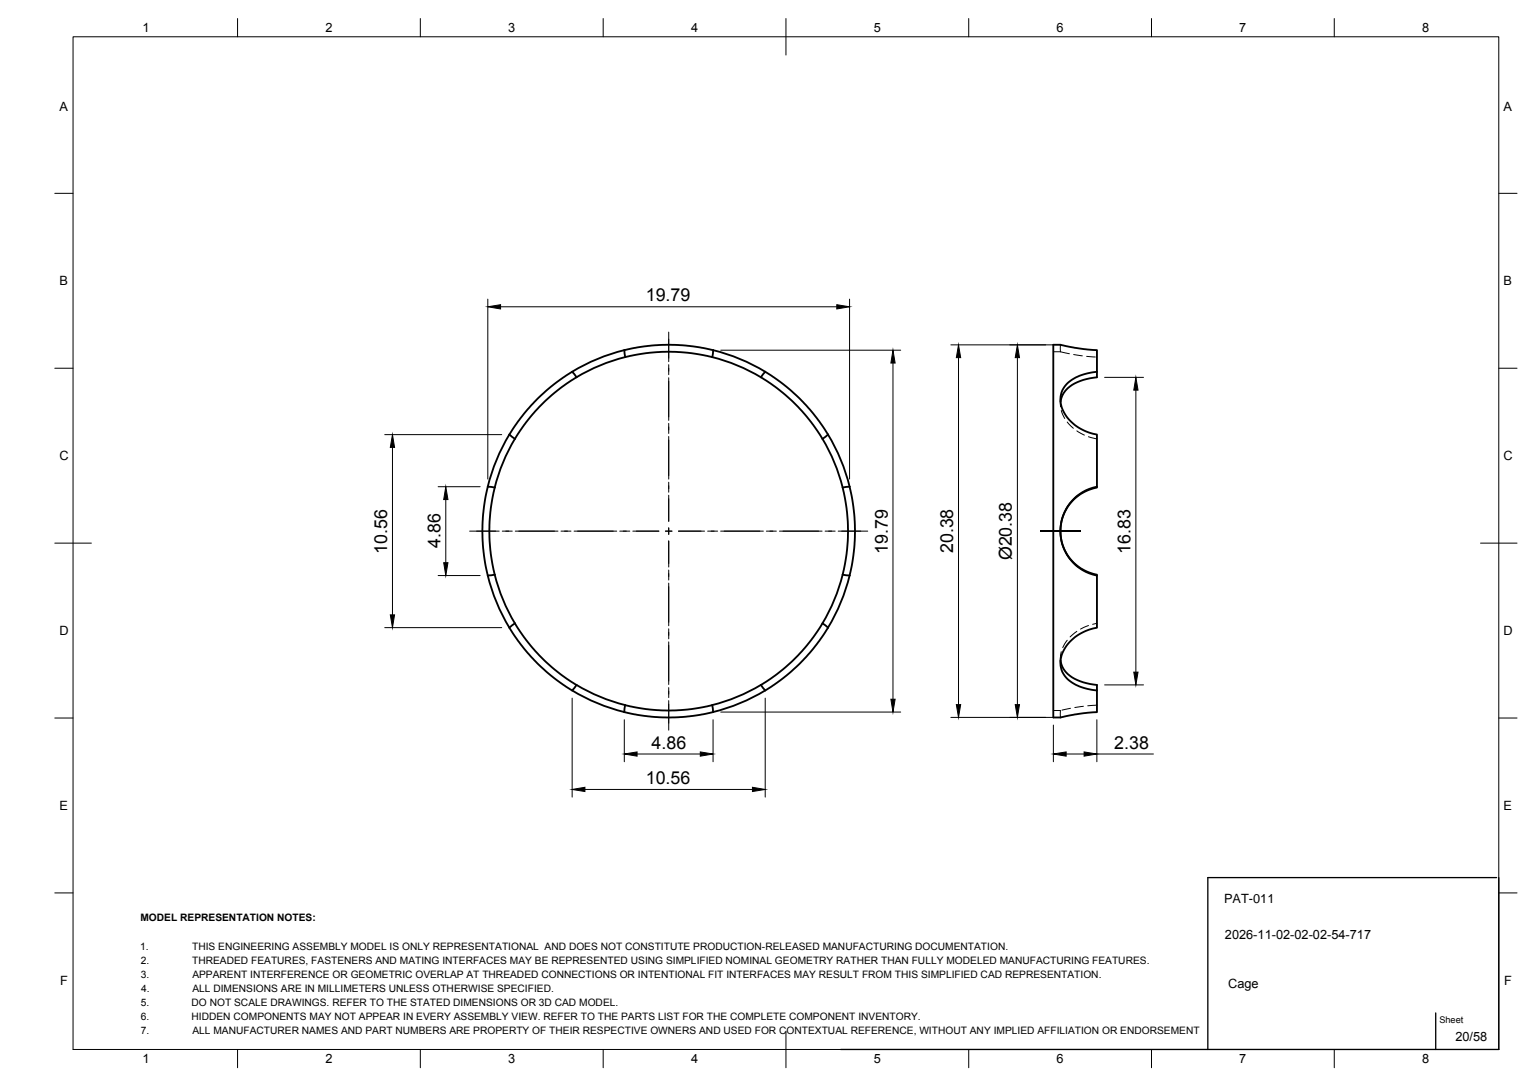
ISO-10303-21;
HEADER;
/* Generated by software containing ST-Developer
 * from STEP Tools, Inc. (www.steptools.com) 
 */

FILE_DESCRIPTION(
/* description */ ('Belt tension measurement rig'),
/* implementation_level */ '2;1');

FILE_NAME(
/* name */ 'Cage.step',
/* time_stamp */ '2026-10-28T03:24:44-07:00',
/* author */ (''),
/* organization */ (''),
/* preprocessor_version */ 'ST-DEVELOPER v20.2',
/* originating_system */ 'Autodesk Translation Framework v15.17.0.0',
/* authorisation */ '');

FILE_SCHEMA (('AUTOMOTIVE_DESIGN { 1 0 10303 214 3 1 1 }'));
ENDSEC;

DATA;
#10=MECHANICAL_DESIGN_GEOMETRIC_PRESENTATION_REPRESENTATION('',(#716),#23587);
#445=SPHERICAL_SURFACE('',#13280,0.247676);
#446=SPHERICAL_SURFACE('',#13296,0.247676);
#447=SPHERICAL_SURFACE('',#13301,0.247676);
#448=SPHERICAL_SURFACE('',#13306,0.247676);
#449=SPHERICAL_SURFACE('',#13311,0.247676);
#450=SPHERICAL_SURFACE('',#13316,0.247676);
#451=SPHERICAL_SURFACE('',#13321,0.247676);
#452=SPHERICAL_SURFACE('',#13329,0.247676);
#495=B_SPLINE_CURVE_WITH_KNOTS('',3,(#19542,#19543,#19544,#19545,#19546,
#19547,#19548,#19549,#19550,#19551,#19552,#19553,#19554,#19555,#19556,#19557,
#19558,#19559,#19560,#19561,#19562,#19563),.UNSPECIFIED.,.F.,.F.,(4,2,2,
2,2,2,2,2,2,2,4),(0.0473477652366656,0.126350602536658,0.189525903804987,
0.252701205073317,0.313298422430275,0.373895639787233,0.434492857144191,
0.495090074501149,0.558265375769478,0.621440677037807,0.7004435143378),
 .UNSPECIFIED.);
#496=B_SPLINE_CURVE_WITH_KNOTS('',3,(#19567,#19568,#19569,#19570,#19571,
#19572,#19573,#19574,#19575,#19576,#19577,#19578,#19579,#19580,#19581,#19582,
#19583,#19584,#19585,#19586,#19587,#19588),.UNSPECIFIED.,.F.,.F.,(4,2,2,
2,2,2,2,2,2,2,4),(0.0464897534940957,0.0852567806515119,0.170513561303024,
0.246687263103517,0.308657850341199,0.370628437578881,0.432599024816563,
0.494569612054245,0.570743313854739,0.656000094506251,0.694767121663666),
 .UNSPECIFIED.);
#497=B_SPLINE_CURVE_WITH_KNOTS('',3,(#19594,#19595,#19596,#19597,#19598,
#19599,#19600,#19601,#19602,#19603,#19604,#19605,#19606,#19607,#19608,#19609,
#19610,#19611,#19612,#19613,#19614,#19615),.UNSPECIFIED.,.F.,.F.,(4,2,2,
2,2,2,2,2,2,2,4),(0.0464897534940957,0.0852567806515118,0.170513561303024,
0.246687263103517,0.308657850341199,0.370628437578881,0.432599024816563,
0.494569612054245,0.570743313854738,0.65600009450625,0.694767121663666),
 .UNSPECIFIED.);
#498=B_SPLINE_CURVE_WITH_KNOTS('',3,(#19619,#19620,#19621,#19622,#19623,
#19624,#19625,#19626,#19627,#19628,#19629,#19630,#19631,#19632,#19633,#19634,
#19635,#19636,#19637,#19638,#19639,#19640),.UNSPECIFIED.,.F.,.F.,(4,2,2,
2,2,2,2,2,2,2,4),(0.0464897534940957,0.0852567806515119,0.170513561303024,
0.246687263103517,0.308657850341199,0.370628437578881,0.432599024816563,
0.494569612054245,0.570743313854739,0.656000094506251,0.694767121663666),
 .UNSPECIFIED.);
#499=B_SPLINE_CURVE_WITH_KNOTS('',3,(#19644,#19645,#19646,#19647,#19648,
#19649,#19650,#19651,#19652,#19653,#19654,#19655),.UNSPECIFIED.,.F.,.F.,
(4,2,2,2,2,4),(0.0464897534940957,0.0852567806515119,0.170513561303024,
0.246687263103517,0.308657850341199,0.370628437578881),.UNSPECIFIED.);
#500=B_SPLINE_CURVE_WITH_KNOTS('',3,(#19660,#19661,#19662,#19663,#19664,
#19665,#19666,#19667,#19668,#19669,#19670,#19671),.UNSPECIFIED.,.F.,.F.,
(4,2,2,2,2,4),(0.370628437578881,0.432599024816563,0.494569612054245,0.570743313854738,
0.65600009450625,0.694767121663666),.UNSPECIFIED.);
#501=B_SPLINE_CURVE_WITH_KNOTS('',3,(#19675,#19676,#19677,#19678,#19679,
#19680,#19681,#19682,#19683,#19684,#19685,#19686,#19687,#19688,#19689,#19690,
#19691,#19692,#19693,#19694,#19695,#19696),.UNSPECIFIED.,.F.,.F.,(4,2,2,
2,2,2,2,2,2,2,4),(0.0464897534940957,0.0852567806515121,0.170513561303024,
0.246687263103518,0.308657850341199,0.370628437578881,0.432599024816563,
0.494569612054245,0.570743313854738,0.65600009450625,0.694767121663666),
 .UNSPECIFIED.);
#502=B_SPLINE_CURVE_WITH_KNOTS('',3,(#19700,#19701,#19702,#19703,#19704,
#19705,#19706,#19707,#19708,#19709,#19710,#19711,#19712,#19713,#19714,#19715,
#19716,#19717,#19718,#19719,#19720,#19721),.UNSPECIFIED.,.F.,.F.,(4,2,2,
2,2,2,2,2,2,2,4),(0.0464897534940957,0.0852567806515119,0.170513561303024,
0.246687263103517,0.308657850341199,0.370628437578881,0.432599024816563,
0.494569612054245,0.570743313854738,0.65600009450625,0.694767121663667),
 .UNSPECIFIED.);
#503=B_SPLINE_CURVE_WITH_KNOTS('',3,(#19725,#19726,#19727,#19728,#19729,
#19730,#19731,#19732,#19733,#19734,#19735,#19736,#19737,#19738,#19739,#19740,
#19741,#19742,#19743,#19744,#19745,#19746),.UNSPECIFIED.,.F.,.F.,(4,2,2,
2,2,2,2,2,2,2,4),(0.0464897534940957,0.0852567806515119,0.170513561303024,
0.246687263103517,0.308657850341199,0.370628437578881,0.432599024816563,
0.494569612054245,0.570743313854738,0.65600009450625,0.694767121663666),
 .UNSPECIFIED.);
#504=B_SPLINE_CURVE_WITH_KNOTS('',3,(#19750,#19751,#19752,#19753,#19754,
#19755,#19756,#19757,#19758,#19759,#19760,#19761,#19762,#19763,#19764,#19765,
#19766,#19767,#19768,#19769,#19770,#19771),.UNSPECIFIED.,.F.,.F.,(4,2,2,
2,2,2,2,2,2,2,4),(0.0464897534940957,0.0852567806515119,0.170513561303024,
0.246687263103517,0.308657850341199,0.370628437578881,0.432599024816563,
0.494569612054245,0.570743313854739,0.656000094506251,0.694767121663667),
 .UNSPECIFIED.);
#505=B_SPLINE_CURVE_WITH_KNOTS('',3,(#19779,#19780,#19781,#19782,#19783,
#19784,#19785,#19786,#19787,#19788,#19789,#19790,#19791,#19792,#19793,#19794,
#19795,#19796,#19797,#19798,#19799,#19800),.UNSPECIFIED.,.F.,.F.,(4,2,2,
2,2,2,2,2,2,2,4),(0.0473477652366656,0.126350602536658,0.189525903804987,
0.252701205073316,0.313298422430274,0.373895639787232,0.434492857144191,
0.495090074501149,0.558265375769478,0.621440677037807,0.7004435143378),
 .UNSPECIFIED.);
#506=B_SPLINE_CURVE_WITH_KNOTS('',3,(#19808,#19809,#19810,#19811,#19812,
#19813,#19814,#19815,#19816,#19817,#19818,#19819,#19820,#19821,#19822,#19823,
#19824,#19825,#19826,#19827,#19828,#19829),.UNSPECIFIED.,.F.,.F.,(4,2,2,
2,2,2,2,2,2,2,4),(0.0473477652366656,0.126350602536658,0.189525903804987,
0.252701205073317,0.313298422430275,0.373895639787233,0.434492857144191,
0.495090074501149,0.558265375769478,0.621440677037807,0.7004435143378),
 .UNSPECIFIED.);
#507=B_SPLINE_CURVE_WITH_KNOTS('',3,(#19838,#19839,#19840,#19841,#19842,
#19843,#19844,#19845,#19846,#19847,#19848,#19849),.UNSPECIFIED.,.F.,.F.,
(4,2,2,2,2,4),(0.0473477652366656,0.126350602536658,0.189525903804987,0.252701205073316,
0.313298422430275,0.373895639787233),.UNSPECIFIED.);
#508=B_SPLINE_CURVE_WITH_KNOTS('',3,(#19851,#19852,#19853,#19854,#19855,
#19856,#19857,#19858,#19859,#19860,#19861,#19862),.UNSPECIFIED.,.F.,.F.,
(4,2,2,2,2,4),(0.373895639787233,0.434492857144191,0.495090074501149,0.558265375769478,
0.621440677037807,0.7004435143378),.UNSPECIFIED.);
#509=B_SPLINE_CURVE_WITH_KNOTS('',3,(#19869,#19870,#19871,#19872,#19873,
#19874,#19875,#19876,#19877,#19878,#19879,#19880,#19881,#19882,#19883,#19884,
#19885,#19886,#19887,#19888,#19889,#19890),.UNSPECIFIED.,.F.,.F.,(4,2,2,
2,2,2,2,2,2,2,4),(0.0473477652366656,0.126350602536658,0.189525903804987,
0.252701205073316,0.313298422430275,0.373895639787233,0.434492857144191,
0.495090074501149,0.558265375769478,0.621440677037807,0.7004435143378),
 .UNSPECIFIED.);
#510=B_SPLINE_CURVE_WITH_KNOTS('',3,(#19898,#19899,#19900,#19901,#19902,
#19903,#19904,#19905,#19906,#19907,#19908,#19909,#19910,#19911,#19912,#19913,
#19914,#19915,#19916,#19917,#19918,#19919),.UNSPECIFIED.,.F.,.F.,(4,2,2,
2,2,2,2,2,2,2,4),(0.0473477652366656,0.126350602536658,0.189525903804987,
0.252701205073317,0.313298422430275,0.373895639787233,0.434492857144191,
0.495090074501149,0.558265375769478,0.621440677037807,0.7004435143378),
 .UNSPECIFIED.);
#511=B_SPLINE_CURVE_WITH_KNOTS('',3,(#19927,#19928,#19929,#19930,#19931,
#19932,#19933,#19934,#19935,#19936,#19937,#19938,#19939,#19940,#19941,#19942,
#19943,#19944,#19945,#19946,#19947,#19948),.UNSPECIFIED.,.F.,.F.,(4,2,2,
2,2,2,2,2,2,2,4),(0.0473477652366656,0.126350602536658,0.189525903804987,
0.252701205073316,0.313298422430275,0.373895639787233,0.434492857144191,
0.495090074501149,0.558265375769478,0.621440677037807,0.7004435143378),
 .UNSPECIFIED.);
#512=B_SPLINE_CURVE_WITH_KNOTS('',3,(#19957,#19958,#19959,#19960,#19961,
#19962,#19963,#19964,#19965,#19966,#19967,#19968,#19969,#19970,#19971,#19972,
#19973,#19974,#19975,#19976,#19977,#19978),.UNSPECIFIED.,.F.,.F.,(4,2,2,
2,2,2,2,2,2,2,4),(0.0473477652366656,0.126350602536658,0.189525903804987,
0.252701205073317,0.313298422430275,0.373895639787233,0.434492857144191,
0.495090074501149,0.558265375769478,0.621440677037807,0.7004435143378),
 .UNSPECIFIED.);
#599=SHAPE_REPRESENTATION_RELATIONSHIP('SRR','None',#23845,#654);
#654=ADVANCED_BREP_SHAPE_REPRESENTATION('',(#786),#23543);
#716=STYLED_ITEM('',(#24211),#786);
#786=MANIFOLD_SOLID_BREP('Continuous crown cage',#12221);
#911=FACE_BOUND('',#2357,.T.);
#1142=PLANE('',#13293);
#1143=PLANE('',#13298);
#1144=PLANE('',#13303);
#1145=PLANE('',#13308);
#1146=PLANE('',#13313);
#1147=PLANE('',#13318);
#1148=PLANE('',#13327);
#1149=PLANE('',#13331);
#1150=PLANE('',#13332);
#1553=FACE_OUTER_BOUND('',#2339,.T.);
#1554=FACE_OUTER_BOUND('',#2340,.T.);
#1555=FACE_OUTER_BOUND('',#2341,.T.);
#1556=FACE_OUTER_BOUND('',#2342,.T.);
#1557=FACE_OUTER_BOUND('',#2343,.T.);
#1558=FACE_OUTER_BOUND('',#2344,.T.);
#1559=FACE_OUTER_BOUND('',#2345,.T.);
#1560=FACE_OUTER_BOUND('',#2346,.T.);
#1561=FACE_OUTER_BOUND('',#2347,.T.);
#1562=FACE_OUTER_BOUND('',#2348,.T.);
#1563=FACE_OUTER_BOUND('',#2349,.T.);
#1564=FACE_OUTER_BOUND('',#2350,.T.);
#1565=FACE_OUTER_BOUND('',#2351,.T.);
#1566=FACE_OUTER_BOUND('',#2352,.T.);
#1567=FACE_OUTER_BOUND('',#2353,.T.);
#1568=FACE_OUTER_BOUND('',#2354,.T.);
#1569=FACE_OUTER_BOUND('',#2355,.T.);
#1570=FACE_OUTER_BOUND('',#2356,.T.);
#1571=FACE_OUTER_BOUND('',#2358,.T.);
#2339=EDGE_LOOP('',(#8764,#8765,#8766,#8767));
#2340=EDGE_LOOP('',(#8768,#8769,#8770,#8771,#8772,#8773,#8774,#8775,#8776,
#8777,#8778,#8779,#8780,#8781,#8782,#8783,#8784,#8785,#8786,#8787));
#2341=EDGE_LOOP('',(#8788,#8789,#8790,#8791));
#2342=EDGE_LOOP('',(#8792,#8793,#8794,#8795));
#2343=EDGE_LOOP('',(#8796,#8797,#8798,#8799));
#2344=EDGE_LOOP('',(#8800,#8801,#8802,#8803));
#2345=EDGE_LOOP('',(#8804,#8805,#8806,#8807));
#2346=EDGE_LOOP('',(#8808,#8809,#8810,#8811,#8812,#8813));
#2347=EDGE_LOOP('',(#8814,#8815,#8816,#8817));
#2348=EDGE_LOOP('',(#8818,#8819,#8820,#8821));
#2349=EDGE_LOOP('',(#8822,#8823,#8824,#8825));
#2350=EDGE_LOOP('',(#8826,#8827,#8828,#8829));
#2351=EDGE_LOOP('',(#8830,#8831,#8832,#8833));
#2352=EDGE_LOOP('',(#8834,#8835,#8836,#8837));
#2353=EDGE_LOOP('',(#8838,#8839,#8840,#8841,#8842,#8843,#8844,#8845,#8846,
#8847,#8848,#8849,#8850,#8851,#8852,#8853,#8854,#8855,#8856,#8857));
#2354=EDGE_LOOP('',(#8858,#8859,#8860,#8861));
#2355=EDGE_LOOP('',(#8862,#8863,#8864,#8865));
#2356=EDGE_LOOP('',(#8866));
#2357=EDGE_LOOP('',(#8867));
#2358=EDGE_LOOP('',(#8868,#8869,#8870,#8871));
#3195=LINE('',#19657,#3946);
#3196=LINE('',#19953,#3947);
#3946=VECTOR('',#15566,1.019052);
#3947=VECTOR('',#15643,0.980948);
#4652=CIRCLE('',#13281,0.243053047864041);
#4653=CIRCLE('',#13282,0.243053047864041);
#4654=CIRCLE('',#13284,1.019052);
#4655=CIRCLE('',#13285,1.019052);
#4656=CIRCLE('',#13286,1.019052);
#4657=CIRCLE('',#13287,1.019052);
#4658=CIRCLE('',#13288,1.019052);
#4659=CIRCLE('',#13289,1.019052);
#4660=CIRCLE('',#13290,1.019052);
#4661=CIRCLE('',#13291,1.019052);
#4662=CIRCLE('',#13292,1.019052);
#4663=CIRCLE('',#13294,0.980948);
#4664=CIRCLE('',#13295,0.243053047864041);
#4665=CIRCLE('',#13297,0.243053047864041);
#4666=CIRCLE('',#13299,0.980948);
#4667=CIRCLE('',#13300,0.243053047864041);
#4668=CIRCLE('',#13302,0.243053047864041);
#4669=CIRCLE('',#13304,0.980948);
#4670=CIRCLE('',#13305,0.243053047864041);
#4671=CIRCLE('',#13307,0.243053047864041);
#4672=CIRCLE('',#13309,0.980948);
#4673=CIRCLE('',#13310,0.243053047864041);
#4674=CIRCLE('',#13312,0.243053047864041);
#4675=CIRCLE('',#13314,0.980948);
#4676=CIRCLE('',#13315,0.243053047864041);
#4677=CIRCLE('',#13317,0.243053047864041);
#4678=CIRCLE('',#13319,0.980948);
#4679=CIRCLE('',#13320,0.243053047864041);
#4680=CIRCLE('',#13322,0.243053047864041);
#4681=CIRCLE('',#13324,0.980948);
#4682=CIRCLE('',#13325,0.980948);
#4683=CIRCLE('',#13326,0.980948);
#4684=CIRCLE('',#13328,0.243053047864041);
#4685=CIRCLE('',#13330,0.243053047864041);
#5520=VERTEX_POINT('',#19540);
#5521=VERTEX_POINT('',#19541);
#5522=VERTEX_POINT('',#19564);
#5523=VERTEX_POINT('',#19566);
#5524=VERTEX_POINT('',#19591);
#5525=VERTEX_POINT('',#19593);
#5526=VERTEX_POINT('',#19616);
#5527=VERTEX_POINT('',#19618);
#5528=VERTEX_POINT('',#19641);
#5529=VERTEX_POINT('',#19643);
#5530=VERTEX_POINT('',#19656);
#5531=VERTEX_POINT('',#19659);
#5532=VERTEX_POINT('',#19672);
#5533=VERTEX_POINT('',#19674);
#5534=VERTEX_POINT('',#19697);
#5535=VERTEX_POINT('',#19699);
#5536=VERTEX_POINT('',#19722);
#5537=VERTEX_POINT('',#19724);
#5538=VERTEX_POINT('',#19747);
#5539=VERTEX_POINT('',#19749);
#5540=VERTEX_POINT('',#19774);
#5541=VERTEX_POINT('',#19778);
#5542=VERTEX_POINT('',#19803);
#5543=VERTEX_POINT('',#19807);
#5544=VERTEX_POINT('',#19832);
#5545=VERTEX_POINT('',#19836);
#5546=VERTEX_POINT('',#19837);
#5547=VERTEX_POINT('',#19864);
#5548=VERTEX_POINT('',#19868);
#5549=VERTEX_POINT('',#19893);
#5550=VERTEX_POINT('',#19897);
#5551=VERTEX_POINT('',#19922);
#5552=VERTEX_POINT('',#19926);
#5553=VERTEX_POINT('',#19951);
#5554=VERTEX_POINT('',#19954);
#5555=VERTEX_POINT('',#19956);
#6741=EDGE_CURVE('',#5520,#5521,#495,.T.);
#6742=EDGE_CURVE('',#5522,#5520,#4652,.T.);
#6743=EDGE_CURVE('',#5523,#5522,#496,.T.);
#6744=EDGE_CURVE('',#5521,#5523,#4653,.T.);
#6745=EDGE_CURVE('',#5524,#5522,#4654,.T.);
#6746=EDGE_CURVE('',#5524,#5525,#497,.T.);
#6747=EDGE_CURVE('',#5526,#5525,#4655,.T.);
#6748=EDGE_CURVE('',#5526,#5527,#498,.T.);
#6749=EDGE_CURVE('',#5528,#5527,#4656,.T.);
#6750=EDGE_CURVE('',#5528,#5529,#499,.T.);
#6751=EDGE_CURVE('',#5529,#5530,#3195,.T.);
#6752=EDGE_CURVE('',#5530,#5530,#4657,.T.);
#6753=EDGE_CURVE('',#5529,#5531,#500,.T.);
#6754=EDGE_CURVE('',#5532,#5531,#4658,.T.);
#6755=EDGE_CURVE('',#5532,#5533,#501,.T.);
#6756=EDGE_CURVE('',#5534,#5533,#4659,.T.);
#6757=EDGE_CURVE('',#5534,#5535,#502,.T.);
#6758=EDGE_CURVE('',#5536,#5535,#4660,.T.);
#6759=EDGE_CURVE('',#5536,#5537,#503,.T.);
#6760=EDGE_CURVE('',#5538,#5537,#4661,.T.);
#6761=EDGE_CURVE('',#5538,#5539,#504,.T.);
#6762=EDGE_CURVE('',#5523,#5539,#4662,.T.);
#6763=EDGE_CURVE('',#5520,#5540,#4663,.T.);
#6764=EDGE_CURVE('',#5540,#5524,#4664,.T.);
#6765=EDGE_CURVE('',#5541,#5540,#505,.T.);
#6766=EDGE_CURVE('',#5525,#5541,#4665,.T.);
#6767=EDGE_CURVE('',#5541,#5542,#4666,.T.);
#6768=EDGE_CURVE('',#5542,#5526,#4667,.T.);
#6769=EDGE_CURVE('',#5543,#5542,#506,.T.);
#6770=EDGE_CURVE('',#5527,#5543,#4668,.T.);
#6771=EDGE_CURVE('',#5543,#5544,#4669,.T.);
#6772=EDGE_CURVE('',#5544,#5528,#4670,.T.);
#6773=EDGE_CURVE('',#5545,#5546,#507,.T.);
#6774=EDGE_CURVE('',#5531,#5545,#4671,.T.);
#6775=EDGE_CURVE('',#5546,#5544,#508,.T.);
#6776=EDGE_CURVE('',#5545,#5547,#4672,.T.);
#6777=EDGE_CURVE('',#5547,#5532,#4673,.T.);
#6778=EDGE_CURVE('',#5548,#5547,#509,.T.);
#6779=EDGE_CURVE('',#5533,#5548,#4674,.T.);
#6780=EDGE_CURVE('',#5548,#5549,#4675,.T.);
#6781=EDGE_CURVE('',#5549,#5534,#4676,.T.);
#6782=EDGE_CURVE('',#5550,#5549,#510,.T.);
#6783=EDGE_CURVE('',#5535,#5550,#4677,.T.);
#6784=EDGE_CURVE('',#5550,#5551,#4678,.T.);
#6785=EDGE_CURVE('',#5551,#5536,#4679,.T.);
#6786=EDGE_CURVE('',#5552,#5551,#511,.T.);
#6787=EDGE_CURVE('',#5537,#5552,#4680,.T.);
#6788=EDGE_CURVE('',#5553,#5553,#4681,.T.);
#6789=EDGE_CURVE('',#5553,#5546,#3196,.T.);
#6790=EDGE_CURVE('',#5554,#5521,#4682,.T.);
#6791=EDGE_CURVE('',#5554,#5555,#512,.T.);
#6792=EDGE_CURVE('',#5552,#5555,#4683,.T.);
#6793=EDGE_CURVE('',#5539,#5554,#4684,.T.);
#6794=EDGE_CURVE('',#5555,#5538,#4685,.T.);
#8764=ORIENTED_EDGE('',*,*,#6741,.F.);
#8765=ORIENTED_EDGE('',*,*,#6742,.F.);
#8766=ORIENTED_EDGE('',*,*,#6743,.F.);
#8767=ORIENTED_EDGE('',*,*,#6744,.F.);
#8768=ORIENTED_EDGE('',*,*,#6743,.T.);
#8769=ORIENTED_EDGE('',*,*,#6745,.F.);
#8770=ORIENTED_EDGE('',*,*,#6746,.T.);
#8771=ORIENTED_EDGE('',*,*,#6747,.F.);
#8772=ORIENTED_EDGE('',*,*,#6748,.T.);
#8773=ORIENTED_EDGE('',*,*,#6749,.F.);
#8774=ORIENTED_EDGE('',*,*,#6750,.T.);
#8775=ORIENTED_EDGE('',*,*,#6751,.T.);
#8776=ORIENTED_EDGE('',*,*,#6752,.F.);
#8777=ORIENTED_EDGE('',*,*,#6751,.F.);
#8778=ORIENTED_EDGE('',*,*,#6753,.T.);
#8779=ORIENTED_EDGE('',*,*,#6754,.F.);
#8780=ORIENTED_EDGE('',*,*,#6755,.T.);
#8781=ORIENTED_EDGE('',*,*,#6756,.F.);
#8782=ORIENTED_EDGE('',*,*,#6757,.T.);
#8783=ORIENTED_EDGE('',*,*,#6758,.F.);
#8784=ORIENTED_EDGE('',*,*,#6759,.T.);
#8785=ORIENTED_EDGE('',*,*,#6760,.F.);
#8786=ORIENTED_EDGE('',*,*,#6761,.T.);
#8787=ORIENTED_EDGE('',*,*,#6762,.F.);
#8788=ORIENTED_EDGE('',*,*,#6742,.T.);
#8789=ORIENTED_EDGE('',*,*,#6763,.T.);
#8790=ORIENTED_EDGE('',*,*,#6764,.T.);
#8791=ORIENTED_EDGE('',*,*,#6745,.T.);
#8792=ORIENTED_EDGE('',*,*,#6765,.F.);
#8793=ORIENTED_EDGE('',*,*,#6766,.F.);
#8794=ORIENTED_EDGE('',*,*,#6746,.F.);
#8795=ORIENTED_EDGE('',*,*,#6764,.F.);
#8796=ORIENTED_EDGE('',*,*,#6766,.T.);
#8797=ORIENTED_EDGE('',*,*,#6767,.T.);
#8798=ORIENTED_EDGE('',*,*,#6768,.T.);
#8799=ORIENTED_EDGE('',*,*,#6747,.T.);
#8800=ORIENTED_EDGE('',*,*,#6769,.F.);
#8801=ORIENTED_EDGE('',*,*,#6770,.F.);
#8802=ORIENTED_EDGE('',*,*,#6748,.F.);
#8803=ORIENTED_EDGE('',*,*,#6768,.F.);
#8804=ORIENTED_EDGE('',*,*,#6770,.T.);
#8805=ORIENTED_EDGE('',*,*,#6771,.T.);
#8806=ORIENTED_EDGE('',*,*,#6772,.T.);
#8807=ORIENTED_EDGE('',*,*,#6749,.T.);
#8808=ORIENTED_EDGE('',*,*,#6773,.F.);
#8809=ORIENTED_EDGE('',*,*,#6774,.F.);
#8810=ORIENTED_EDGE('',*,*,#6753,.F.);
#8811=ORIENTED_EDGE('',*,*,#6750,.F.);
#8812=ORIENTED_EDGE('',*,*,#6772,.F.);
#8813=ORIENTED_EDGE('',*,*,#6775,.F.);
#8814=ORIENTED_EDGE('',*,*,#6774,.T.);
#8815=ORIENTED_EDGE('',*,*,#6776,.T.);
#8816=ORIENTED_EDGE('',*,*,#6777,.T.);
#8817=ORIENTED_EDGE('',*,*,#6754,.T.);
#8818=ORIENTED_EDGE('',*,*,#6778,.F.);
#8819=ORIENTED_EDGE('',*,*,#6779,.F.);
#8820=ORIENTED_EDGE('',*,*,#6755,.F.);
#8821=ORIENTED_EDGE('',*,*,#6777,.F.);
#8822=ORIENTED_EDGE('',*,*,#6779,.T.);
#8823=ORIENTED_EDGE('',*,*,#6780,.T.);
#8824=ORIENTED_EDGE('',*,*,#6781,.T.);
#8825=ORIENTED_EDGE('',*,*,#6756,.T.);
#8826=ORIENTED_EDGE('',*,*,#6782,.F.);
#8827=ORIENTED_EDGE('',*,*,#6783,.F.);
#8828=ORIENTED_EDGE('',*,*,#6757,.F.);
#8829=ORIENTED_EDGE('',*,*,#6781,.F.);
#8830=ORIENTED_EDGE('',*,*,#6783,.T.);
#8831=ORIENTED_EDGE('',*,*,#6784,.T.);
#8832=ORIENTED_EDGE('',*,*,#6785,.T.);
#8833=ORIENTED_EDGE('',*,*,#6758,.T.);
#8834=ORIENTED_EDGE('',*,*,#6759,.F.);
#8835=ORIENTED_EDGE('',*,*,#6785,.F.);
#8836=ORIENTED_EDGE('',*,*,#6786,.F.);
#8837=ORIENTED_EDGE('',*,*,#6787,.F.);
#8838=ORIENTED_EDGE('',*,*,#6788,.F.);
#8839=ORIENTED_EDGE('',*,*,#6789,.T.);
#8840=ORIENTED_EDGE('',*,*,#6775,.T.);
#8841=ORIENTED_EDGE('',*,*,#6771,.F.);
#8842=ORIENTED_EDGE('',*,*,#6769,.T.);
#8843=ORIENTED_EDGE('',*,*,#6767,.F.);
#8844=ORIENTED_EDGE('',*,*,#6765,.T.);
#8845=ORIENTED_EDGE('',*,*,#6763,.F.);
#8846=ORIENTED_EDGE('',*,*,#6741,.T.);
#8847=ORIENTED_EDGE('',*,*,#6790,.F.);
#8848=ORIENTED_EDGE('',*,*,#6791,.T.);
#8849=ORIENTED_EDGE('',*,*,#6792,.F.);
#8850=ORIENTED_EDGE('',*,*,#6786,.T.);
#8851=ORIENTED_EDGE('',*,*,#6784,.F.);
#8852=ORIENTED_EDGE('',*,*,#6782,.T.);
#8853=ORIENTED_EDGE('',*,*,#6780,.F.);
#8854=ORIENTED_EDGE('',*,*,#6778,.T.);
#8855=ORIENTED_EDGE('',*,*,#6776,.F.);
#8856=ORIENTED_EDGE('',*,*,#6773,.T.);
#8857=ORIENTED_EDGE('',*,*,#6789,.F.);
#8858=ORIENTED_EDGE('',*,*,#6744,.T.);
#8859=ORIENTED_EDGE('',*,*,#6762,.T.);
#8860=ORIENTED_EDGE('',*,*,#6793,.T.);
#8861=ORIENTED_EDGE('',*,*,#6790,.T.);
#8862=ORIENTED_EDGE('',*,*,#6761,.F.);
#8863=ORIENTED_EDGE('',*,*,#6794,.F.);
#8864=ORIENTED_EDGE('',*,*,#6791,.F.);
#8865=ORIENTED_EDGE('',*,*,#6793,.F.);
#8866=ORIENTED_EDGE('',*,*,#6752,.T.);
#8867=ORIENTED_EDGE('',*,*,#6788,.T.);
#8868=ORIENTED_EDGE('',*,*,#6787,.T.);
#8869=ORIENTED_EDGE('',*,*,#6792,.T.);
#8870=ORIENTED_EDGE('',*,*,#6794,.T.);
#8871=ORIENTED_EDGE('',*,*,#6760,.T.);
#11240=CYLINDRICAL_SURFACE('',#13283,1.019052);
#11241=CYLINDRICAL_SURFACE('',#13323,0.980948);
#11694=ADVANCED_FACE('',(#1553),#445,.F.);
#11695=ADVANCED_FACE('',(#1554),#11240,.T.);
#11696=ADVANCED_FACE('',(#1555),#1142,.T.);
#11697=ADVANCED_FACE('',(#1556),#446,.F.);
#11698=ADVANCED_FACE('',(#1557),#1143,.T.);
#11699=ADVANCED_FACE('',(#1558),#447,.F.);
#11700=ADVANCED_FACE('',(#1559),#1144,.T.);
#11701=ADVANCED_FACE('',(#1560),#448,.F.);
#11702=ADVANCED_FACE('',(#1561),#1145,.T.);
#11703=ADVANCED_FACE('',(#1562),#449,.F.);
#11704=ADVANCED_FACE('',(#1563),#1146,.T.);
#11705=ADVANCED_FACE('',(#1564),#450,.F.);
#11706=ADVANCED_FACE('',(#1565),#1147,.T.);
#11707=ADVANCED_FACE('',(#1566),#451,.F.);
#11708=ADVANCED_FACE('',(#1567),#11241,.F.);
#11709=ADVANCED_FACE('',(#1568),#1148,.T.);
#11710=ADVANCED_FACE('',(#1569),#452,.F.);
#11711=ADVANCED_FACE('',(#1570,#911),#1149,.T.);
#11712=ADVANCED_FACE('',(#1571),#1150,.T.);
#12221=CLOSED_SHELL('',(#11694,#11695,#11696,#11697,#11698,#11699,#11700,
#11701,#11702,#11703,#11704,#11705,#11706,#11707,#11708,#11709,#11710,#11711,
#11712));
#13279=AXIS2_PLACEMENT_3D('',#19538,#15550,#15551);
#13280=AXIS2_PLACEMENT_3D('',#19539,#15552,#15553);
#13281=AXIS2_PLACEMENT_3D('',#19565,#15554,#15555);
#13282=AXIS2_PLACEMENT_3D('',#19589,#15556,#15557);
#13283=AXIS2_PLACEMENT_3D('',#19590,#15558,#15559);
#13284=AXIS2_PLACEMENT_3D('',#19592,#15560,#15561);
#13285=AXIS2_PLACEMENT_3D('',#19617,#15562,#15563);
#13286=AXIS2_PLACEMENT_3D('',#19642,#15564,#15565);
#13287=AXIS2_PLACEMENT_3D('',#19658,#15567,#15568);
#13288=AXIS2_PLACEMENT_3D('',#19673,#15569,#15570);
#13289=AXIS2_PLACEMENT_3D('',#19698,#15571,#15572);
#13290=AXIS2_PLACEMENT_3D('',#19723,#15573,#15574);
#13291=AXIS2_PLACEMENT_3D('',#19748,#15575,#15576);
#13292=AXIS2_PLACEMENT_3D('',#19772,#15577,#15578);
#13293=AXIS2_PLACEMENT_3D('',#19773,#15579,#15580);
#13294=AXIS2_PLACEMENT_3D('',#19775,#15581,#15582);
#13295=AXIS2_PLACEMENT_3D('',#19776,#15583,#15584);
#13296=AXIS2_PLACEMENT_3D('',#19777,#15585,#15586);
#13297=AXIS2_PLACEMENT_3D('',#19801,#15587,#15588);
#13298=AXIS2_PLACEMENT_3D('',#19802,#15589,#15590);
#13299=AXIS2_PLACEMENT_3D('',#19804,#15591,#15592);
#13300=AXIS2_PLACEMENT_3D('',#19805,#15593,#15594);
#13301=AXIS2_PLACEMENT_3D('',#19806,#15595,#15596);
#13302=AXIS2_PLACEMENT_3D('',#19830,#15597,#15598);
#13303=AXIS2_PLACEMENT_3D('',#19831,#15599,#15600);
#13304=AXIS2_PLACEMENT_3D('',#19833,#15601,#15602);
#13305=AXIS2_PLACEMENT_3D('',#19834,#15603,#15604);
#13306=AXIS2_PLACEMENT_3D('',#19835,#15605,#15606);
#13307=AXIS2_PLACEMENT_3D('',#19850,#15607,#15608);
#13308=AXIS2_PLACEMENT_3D('',#19863,#15609,#15610);
#13309=AXIS2_PLACEMENT_3D('',#19865,#15611,#15612);
#13310=AXIS2_PLACEMENT_3D('',#19866,#15613,#15614);
#13311=AXIS2_PLACEMENT_3D('',#19867,#15615,#15616);
#13312=AXIS2_PLACEMENT_3D('',#19891,#15617,#15618);
#13313=AXIS2_PLACEMENT_3D('',#19892,#15619,#15620);
#13314=AXIS2_PLACEMENT_3D('',#19894,#15621,#15622);
#13315=AXIS2_PLACEMENT_3D('',#19895,#15623,#15624);
#13316=AXIS2_PLACEMENT_3D('',#19896,#15625,#15626);
#13317=AXIS2_PLACEMENT_3D('',#19920,#15627,#15628);
#13318=AXIS2_PLACEMENT_3D('',#19921,#15629,#15630);
#13319=AXIS2_PLACEMENT_3D('',#19923,#15631,#15632);
#13320=AXIS2_PLACEMENT_3D('',#19924,#15633,#15634);
#13321=AXIS2_PLACEMENT_3D('',#19925,#15635,#15636);
#13322=AXIS2_PLACEMENT_3D('',#19949,#15637,#15638);
#13323=AXIS2_PLACEMENT_3D('',#19950,#15639,#15640);
#13324=AXIS2_PLACEMENT_3D('',#19952,#15641,#15642);
#13325=AXIS2_PLACEMENT_3D('',#19955,#15644,#15645);
#13326=AXIS2_PLACEMENT_3D('',#19979,#15646,#15647);
#13327=AXIS2_PLACEMENT_3D('',#19980,#15648,#15649);
#13328=AXIS2_PLACEMENT_3D('',#19981,#15650,#15651);
#13329=AXIS2_PLACEMENT_3D('',#19982,#15652,#15653);
#13330=AXIS2_PLACEMENT_3D('',#19983,#15654,#15655);
#13331=AXIS2_PLACEMENT_3D('',#19984,#15656,#15657);
#13332=AXIS2_PLACEMENT_3D('',#19985,#15658,#15659);
#15550=DIRECTION('axis',(0.,0.,1.));
#15551=DIRECTION('refdir',(1.,0.,0.));
#15552=DIRECTION('center_axis',(0.,0.,1.));
#15553=DIRECTION('ref_axis',(1.,0.,0.));
#15554=DIRECTION('center_axis',(0.,-1.,0.));
#15555=DIRECTION('ref_axis',(0.,0.,-1.));
#15556=DIRECTION('center_axis',(0.,-1.,0.));
#15557=DIRECTION('ref_axis',(0.,0.,-1.));
#15558=DIRECTION('center_axis',(0.,1.,0.));
#15559=DIRECTION('ref_axis',(1.,0.,0.));
#15560=DIRECTION('center_axis',(0.,1.,0.));
#15561=DIRECTION('ref_axis',(1.,0.,0.));
#15562=DIRECTION('center_axis',(0.,1.,0.));
#15563=DIRECTION('ref_axis',(1.,0.,0.));
#15564=DIRECTION('center_axis',(0.,1.,0.));
#15565=DIRECTION('ref_axis',(1.,0.,0.));
#15566=DIRECTION('',(0.,-1.,0.));
#15567=DIRECTION('center_axis',(0.,-1.,0.));
#15568=DIRECTION('ref_axis',(1.,0.,0.));
#15569=DIRECTION('center_axis',(0.,1.,0.));
#15570=DIRECTION('ref_axis',(1.,0.,0.));
#15571=DIRECTION('center_axis',(0.,1.,0.));
#15572=DIRECTION('ref_axis',(1.,0.,0.));
#15573=DIRECTION('center_axis',(0.,1.,0.));
#15574=DIRECTION('ref_axis',(1.,0.,0.));
#15575=DIRECTION('center_axis',(0.,1.,0.));
#15576=DIRECTION('ref_axis',(1.,0.,0.));
#15577=DIRECTION('center_axis',(0.,1.,0.));
#15578=DIRECTION('ref_axis',(1.,0.,0.));
#15579=DIRECTION('center_axis',(0.,1.,0.));
#15580=DIRECTION('ref_axis',(1.,0.,0.));
#15581=DIRECTION('center_axis',(0.,-1.,0.));
#15582=DIRECTION('ref_axis',(1.,0.,0.));
#15583=DIRECTION('center_axis',(0.,-1.,0.));
#15584=DIRECTION('ref_axis',(0.,0.,-1.));
#15585=DIRECTION('center_axis',(6.12323399573677E-17,0.,1.));
#15586=DIRECTION('ref_axis',(1.,0.,0.));
#15587=DIRECTION('center_axis',(0.,-1.,0.));
#15588=DIRECTION('ref_axis',(0.,0.,-1.));
#15589=DIRECTION('center_axis',(0.,1.,0.));
#15590=DIRECTION('ref_axis',(1.,0.,0.));
#15591=DIRECTION('center_axis',(0.,-1.,0.));
#15592=DIRECTION('ref_axis',(1.,0.,0.));
#15593=DIRECTION('center_axis',(0.,-1.,0.));
#15594=DIRECTION('ref_axis',(0.,0.,-1.));
#15595=DIRECTION('center_axis',(0.,0.,1.));
#15596=DIRECTION('ref_axis',(1.,0.,0.));
#15597=DIRECTION('center_axis',(0.,-1.,0.));
#15598=DIRECTION('ref_axis',(0.,0.,-1.));
#15599=DIRECTION('center_axis',(0.,1.,0.));
#15600=DIRECTION('ref_axis',(1.,0.,0.));
#15601=DIRECTION('center_axis',(0.,-1.,0.));
#15602=DIRECTION('ref_axis',(1.,0.,0.));
#15603=DIRECTION('center_axis',(0.,-1.,0.));
#15604=DIRECTION('ref_axis',(0.,0.,-1.));
#15605=DIRECTION('center_axis',(0.,0.,1.));
#15606=DIRECTION('ref_axis',(1.,0.,0.));
#15607=DIRECTION('center_axis',(0.,-1.,0.));
#15608=DIRECTION('ref_axis',(0.,0.,-1.));
#15609=DIRECTION('center_axis',(0.,1.,0.));
#15610=DIRECTION('ref_axis',(1.,0.,0.));
#15611=DIRECTION('center_axis',(0.,-1.,0.));
#15612=DIRECTION('ref_axis',(1.,0.,0.));
#15613=DIRECTION('center_axis',(0.,-1.,0.));
#15614=DIRECTION('ref_axis',(0.,0.,-1.));
#15615=DIRECTION('center_axis',(0.,0.,1.));
#15616=DIRECTION('ref_axis',(1.,0.,0.));
#15617=DIRECTION('center_axis',(0.,-1.,0.));
#15618=DIRECTION('ref_axis',(0.,0.,-1.));
#15619=DIRECTION('center_axis',(0.,1.,0.));
#15620=DIRECTION('ref_axis',(1.,0.,0.));
#15621=DIRECTION('center_axis',(0.,-1.,0.));
#15622=DIRECTION('ref_axis',(1.,0.,0.));
#15623=DIRECTION('center_axis',(0.,-1.,0.));
#15624=DIRECTION('ref_axis',(0.,0.,-1.));
#15625=DIRECTION('center_axis',(6.12323399573676E-17,0.,1.));
#15626=DIRECTION('ref_axis',(1.,0.,0.));
#15627=DIRECTION('center_axis',(0.,-1.,0.));
#15628=DIRECTION('ref_axis',(0.,0.,-1.));
#15629=DIRECTION('center_axis',(0.,1.,0.));
#15630=DIRECTION('ref_axis',(1.,0.,0.));
#15631=DIRECTION('center_axis',(0.,-1.,0.));
#15632=DIRECTION('ref_axis',(1.,0.,0.));
#15633=DIRECTION('center_axis',(0.,-1.,0.));
#15634=DIRECTION('ref_axis',(0.,0.,-1.));
#15635=DIRECTION('center_axis',(0.,0.,1.));
#15636=DIRECTION('ref_axis',(1.,0.,0.));
#15637=DIRECTION('center_axis',(0.,-1.,0.));
#15638=DIRECTION('ref_axis',(0.,0.,-1.));
#15639=DIRECTION('center_axis',(0.,1.,0.));
#15640=DIRECTION('ref_axis',(1.,0.,0.));
#15641=DIRECTION('center_axis',(0.,1.,0.));
#15642=DIRECTION('ref_axis',(1.,0.,0.));
#15643=DIRECTION('',(0.,1.,0.));
#15644=DIRECTION('center_axis',(0.,-1.,0.));
#15645=DIRECTION('ref_axis',(1.,0.,0.));
#15646=DIRECTION('center_axis',(0.,-1.,0.));
#15647=DIRECTION('ref_axis',(1.,0.,0.));
#15648=DIRECTION('center_axis',(0.,1.,0.));
#15649=DIRECTION('ref_axis',(1.,0.,0.));
#15650=DIRECTION('center_axis',(0.,-1.,0.));
#15651=DIRECTION('ref_axis',(0.,0.,-1.));
#15652=DIRECTION('center_axis',(0.,0.,1.));
#15653=DIRECTION('ref_axis',(1.,0.,0.));
#15654=DIRECTION('center_axis',(0.,-1.,0.));
#15655=DIRECTION('ref_axis',(0.,0.,-1.));
#15656=DIRECTION('center_axis',(0.,-1.,0.));
#15657=DIRECTION('ref_axis',(-1.,0.,0.));
#15658=DIRECTION('center_axis',(0.,1.,0.));
#15659=DIRECTION('ref_axis',(1.,0.,0.));
#19538=CARTESIAN_POINT('',(0.,0.,0.));
#19539=CARTESIAN_POINT('Origin',(0.707106781186547,0.,0.707106781186548));
#19540=CARTESIAN_POINT('',(0.504455939115715,-0.04763,0.841298510752802));
#19541=CARTESIAN_POINT('',(0.841298510752802,-0.04763,0.504455939115715));
#19542=CARTESIAN_POINT('Ctrl Pts',(0.504455939115715,-0.04763,0.841298510752802));
#19543=CARTESIAN_POINT('Ctrl Pts',(0.508899795931835,-0.0740444353928835,
0.838633903678357));
#19544=CARTESIAN_POINT('Ctrl Pts',(0.517157748491652,-0.0999305678883309,
0.833661031856294));
#19545=CARTESIAN_POINT('Ctrl Pts',(0.537715343527944,-0.142345102874864,
0.820511285096538));
#19546=CARTESIAN_POINT('Ctrl Pts',(0.548874290046456,-0.159766064500479,
0.813159949759));
#19547=CARTESIAN_POINT('Ctrl Pts',(0.573915184558107,-0.190326085855194,
0.795684265985089));
#19548=CARTESIAN_POINT('Ctrl Pts',(0.587792702767295,-0.203463743702801,
0.78555112003688));
#19549=CARTESIAN_POINT('Ctrl Pts',(0.615966552324775,-0.224161999508995,
0.763642258217233));
#19550=CARTESIAN_POINT('Ctrl Pts',(0.631684198665438,-0.232861760990032,
0.750785745543687));
#19551=CARTESIAN_POINT('Ctrl Pts',(0.663382628119203,-0.244251601209411,
0.722929908501543));
#19552=CARTESIAN_POINT('Ctrl Pts',(0.679352081686668,-0.246942143572133,
0.707917883896095));
#19553=CARTESIAN_POINT('Ctrl Pts',(0.707917883896095,-0.246942143572133,
0.679352081686668));
#19554=CARTESIAN_POINT('Ctrl Pts',(0.722929908501543,-0.244251601209411,
0.663382628119203));
#19555=CARTESIAN_POINT('Ctrl Pts',(0.750785745543687,-0.232861760990032,
0.631684198665439));
#19556=CARTESIAN_POINT('Ctrl Pts',(0.763642258217232,-0.224161999508995,
0.615966552324775));
#19557=CARTESIAN_POINT('Ctrl Pts',(0.78555112003688,-0.203463743702801,
0.587792702767295));
#19558=CARTESIAN_POINT('Ctrl Pts',(0.795684265985088,-0.190326085855194,
0.573915184558108));
#19559=CARTESIAN_POINT('Ctrl Pts',(0.813159949759,-0.15976606450048,0.548874290046456));
#19560=CARTESIAN_POINT('Ctrl Pts',(0.820511285096538,-0.142345102874864,
0.537715343527944));
#19561=CARTESIAN_POINT('Ctrl Pts',(0.833661031856294,-0.099930567888331,
0.517157748491653));
#19562=CARTESIAN_POINT('Ctrl Pts',(0.838633903678357,-0.0740444353928835,
0.508899795931835));
#19563=CARTESIAN_POINT('Ctrl Pts',(0.841298510752801,-0.0476299999999999,
0.504455939115715));
#19564=CARTESIAN_POINT('',(0.528110872004958,-0.04763,0.871530771444223));
#19565=CARTESIAN_POINT('Origin',(0.707106781186547,-0.04763,0.707106781186548));
#19566=CARTESIAN_POINT('',(0.871530771444223,-0.04763,0.528110872004959));
#19567=CARTESIAN_POINT('Ctrl Pts',(0.871530771444223,-0.0476300000000001,
0.528110872004958));
#19568=CARTESIAN_POINT('Ctrl Pts',(0.87014664509073,-0.0609922781173483,
0.530395067942936));
#19569=CARTESIAN_POINT('Ctrl Pts',(0.868149331745851,-0.0742967091364493,
0.533674141594226));
#19570=CARTESIAN_POINT('Ctrl Pts',(0.85981294420286,-0.115492077056649,
0.54708917182331));
#19571=CARTESIAN_POINT('Ctrl Pts',(0.850993704737257,-0.141695629206859,
0.560922177770136));
#19572=CARTESIAN_POINT('Ctrl Pts',(0.830754510485543,-0.181890537957859,
0.590422647829571));
#19573=CARTESIAN_POINT('Ctrl Pts',(0.816896541396381,-0.201072148666545,
0.609616703125488));
#19574=CARTESIAN_POINT('Ctrl Pts',(0.792310597819928,-0.223955109275652,
0.641117951819998));
#19575=CARTESIAN_POINT('Ctrl Pts',(0.779109323683612,-0.232742381310829,
0.657208095763053));
#19576=CARTESIAN_POINT('Ctrl Pts',(0.750552691816206,-0.244234834628584,
0.68964083160521));
#19577=CARTESIAN_POINT('Ctrl Pts',(0.735185187071673,-0.246942143572133,
0.705971972091755));
#19578=CARTESIAN_POINT('Ctrl Pts',(0.705971972091754,-0.246942143572133,
0.735185187071673));
#19579=CARTESIAN_POINT('Ctrl Pts',(0.689640831605209,-0.244234834628584,
0.750552691816206));
#19580=CARTESIAN_POINT('Ctrl Pts',(0.657208095763052,-0.232742381310829,
0.779109323683612));
#19581=CARTESIAN_POINT('Ctrl Pts',(0.641117951819998,-0.223955109275652,
0.792310597819928));
#19582=CARTESIAN_POINT('Ctrl Pts',(0.609616703125487,-0.201072148666545,
0.816896541396382));
#19583=CARTESIAN_POINT('Ctrl Pts',(0.590422647829571,-0.181890537957858,
0.830754510485544));
#19584=CARTESIAN_POINT('Ctrl Pts',(0.560922177770135,-0.141695629206858,
0.850993704737257));
#19585=CARTESIAN_POINT('Ctrl Pts',(0.547089171823309,-0.115492077056649,
0.859812944202861));
#19586=CARTESIAN_POINT('Ctrl Pts',(0.533674141594226,-0.0742967091364491,
0.868149331745852));
#19587=CARTESIAN_POINT('Ctrl Pts',(0.530395067942936,-0.0609922781173483,
0.870146645090731));
#19588=CARTESIAN_POINT('Ctrl Pts',(0.528110872004958,-0.0476300000000001,
0.871530771444223));
#19589=CARTESIAN_POINT('Origin',(0.707106781186547,-0.04763,0.707106781186548));
#19590=CARTESIAN_POINT('Origin',(0.,-0.166705,0.));
#19591=CARTESIAN_POINT('',(0.242834539687906,-0.04763,0.989696097314));
#19592=CARTESIAN_POINT('Origin',(0.,-0.04763,0.));
#19593=CARTESIAN_POINT('',(-0.242834539687907,-0.04763,0.989696097314));
#19594=CARTESIAN_POINT('Ctrl Pts',(0.242834539687906,-0.04763,0.989696097314));
#19595=CARTESIAN_POINT('Ctrl Pts',(0.24024064412003,-0.0609922781173483,
0.990332542620729));
#19596=CARTESIAN_POINT('Ctrl Pts',(0.236509675094874,-0.0742967091364492,
0.991238884025248));
#19597=CARTESIAN_POINT('Ctrl Pts',(0.221129100087819,-0.115492077056649,
0.994830026707808));
#19598=CARTESIAN_POINT('Ctrl Pts',(0.205111543747588,-0.141695629206859,
0.998375294985966));
#19599=CARTESIAN_POINT('Ctrl Pts',(0.169940289819232,-0.181890537957859,
1.00492400591205));
#19600=CARTESIAN_POINT('Ctrl Pts',(0.1465689792446,-0.201072148666545,1.00869718865384));
#19601=CARTESIAN_POINT('Ctrl Pts',(0.106909345252087,-0.223955109275652,
1.01358704779679));
#19602=CARTESIAN_POINT('Ctrl Pts',(0.0861971848975941,-0.232742381310829,
1.0156297872271));
#19603=CARTESIAN_POINT('Ctrl Pts',(0.0430711894098822,-0.244234834628584,
1.01837060663223));
#19604=CARTESIAN_POINT('Ctrl Pts',(0.0206568624125605,-0.246942143572133,
1.019052));
#19605=CARTESIAN_POINT('Ctrl Pts',(-0.0206568624125608,-0.246942143572133,
1.019052));
#19606=CARTESIAN_POINT('Ctrl Pts',(-0.0430711894098825,-0.244234834628584,
1.01837060663223));
#19607=CARTESIAN_POINT('Ctrl Pts',(-0.0861971848975943,-0.232742381310829,
1.0156297872271));
#19608=CARTESIAN_POINT('Ctrl Pts',(-0.106909345252088,-0.223955109275652,
1.01358704779679));
#19609=CARTESIAN_POINT('Ctrl Pts',(-0.1465689792446,-0.201072148666545,
1.00869718865384));
#19610=CARTESIAN_POINT('Ctrl Pts',(-0.169940289819232,-0.181890537957859,
1.00492400591205));
#19611=CARTESIAN_POINT('Ctrl Pts',(-0.205111543747588,-0.141695629206859,
0.998375294985966));
#19612=CARTESIAN_POINT('Ctrl Pts',(-0.221129100087819,-0.115492077056649,
0.994830026707808));
#19613=CARTESIAN_POINT('Ctrl Pts',(-0.236509675094875,-0.0742967091364493,
0.991238884025248));
#19614=CARTESIAN_POINT('Ctrl Pts',(-0.24024064412003,-0.0609922781173483,
0.990332542620729));
#19615=CARTESIAN_POINT('Ctrl Pts',(-0.242834539687907,-0.04763,0.989696097314));
#19616=CARTESIAN_POINT('',(-0.528110872004959,-0.04763,0.871530771444223));
#19617=CARTESIAN_POINT('Origin',(0.,-0.04763,0.));
#19618=CARTESIAN_POINT('',(-0.871530771444223,-0.04763,0.528110872004958));
#19619=CARTESIAN_POINT('Ctrl Pts',(-0.528110872004958,-0.0476300000000001,
0.871530771444223));
#19620=CARTESIAN_POINT('Ctrl Pts',(-0.530395067942936,-0.0609922781173484,
0.87014664509073));
#19621=CARTESIAN_POINT('Ctrl Pts',(-0.533674141594226,-0.0742967091364493,
0.868149331745851));
#19622=CARTESIAN_POINT('Ctrl Pts',(-0.54708917182331,-0.115492077056649,
0.85981294420286));
#19623=CARTESIAN_POINT('Ctrl Pts',(-0.560922177770136,-0.141695629206859,
0.850993704737257));
#19624=CARTESIAN_POINT('Ctrl Pts',(-0.590422647829571,-0.181890537957859,
0.830754510485543));
#19625=CARTESIAN_POINT('Ctrl Pts',(-0.609616703125488,-0.201072148666545,
0.816896541396381));
#19626=CARTESIAN_POINT('Ctrl Pts',(-0.641117951819998,-0.223955109275652,
0.792310597819928));
#19627=CARTESIAN_POINT('Ctrl Pts',(-0.657208095763053,-0.232742381310829,
0.779109323683611));
#19628=CARTESIAN_POINT('Ctrl Pts',(-0.68964083160521,-0.244234834628584,
0.750552691816205));
#19629=CARTESIAN_POINT('Ctrl Pts',(-0.705971972091755,-0.246942143572133,
0.735185187071673));
#19630=CARTESIAN_POINT('Ctrl Pts',(-0.735185187071673,-0.246942143572133,
0.705971972091754));
#19631=CARTESIAN_POINT('Ctrl Pts',(-0.750552691816206,-0.244234834628584,
0.689640831605209));
#19632=CARTESIAN_POINT('Ctrl Pts',(-0.779109323683612,-0.232742381310829,
0.657208095763052));
#19633=CARTESIAN_POINT('Ctrl Pts',(-0.792310597819928,-0.223955109275652,
0.641117951819998));
#19634=CARTESIAN_POINT('Ctrl Pts',(-0.816896541396382,-0.201072148666545,
0.609616703125487));
#19635=CARTESIAN_POINT('Ctrl Pts',(-0.830754510485544,-0.181890537957858,
0.590422647829571));
#19636=CARTESIAN_POINT('Ctrl Pts',(-0.850993704737257,-0.141695629206858,
0.560922177770135));
#19637=CARTESIAN_POINT('Ctrl Pts',(-0.859812944202861,-0.115492077056649,
0.547089171823309));
#19638=CARTESIAN_POINT('Ctrl Pts',(-0.868149331745852,-0.0742967091364491,
0.533674141594226));
#19639=CARTESIAN_POINT('Ctrl Pts',(-0.870146645090731,-0.0609922781173483,
0.530395067942936));
#19640=CARTESIAN_POINT('Ctrl Pts',(-0.871530771444223,-0.04763,0.528110872004958));
#19641=CARTESIAN_POINT('',(-0.989696097314,-0.04763,0.242834539687906));
#19642=CARTESIAN_POINT('Origin',(0.,-0.04763,0.));
#19643=CARTESIAN_POINT('',(-1.019052,-0.246942143572133,1.248489836334E-16));
#19644=CARTESIAN_POINT('Ctrl Pts',(-0.989696097314,-0.04763,0.242834539687906));
#19645=CARTESIAN_POINT('Ctrl Pts',(-0.990332542620729,-0.0609922781173483,
0.24024064412003));
#19646=CARTESIAN_POINT('Ctrl Pts',(-0.991238884025248,-0.0742967091364492,
0.236509675094874));
#19647=CARTESIAN_POINT('Ctrl Pts',(-0.994830026707808,-0.115492077056649,
0.221129100087819));
#19648=CARTESIAN_POINT('Ctrl Pts',(-0.998375294985966,-0.141695629206859,
0.205111543747588));
#19649=CARTESIAN_POINT('Ctrl Pts',(-1.00492400591205,-0.181890537957859,
0.169940289819232));
#19650=CARTESIAN_POINT('Ctrl Pts',(-1.00869718865384,-0.201072148666545,
0.1465689792446));
#19651=CARTESIAN_POINT('Ctrl Pts',(-1.01358704779679,-0.223955109275652,
0.106909345252088));
#19652=CARTESIAN_POINT('Ctrl Pts',(-1.0156297872271,-0.232742381310829,
0.0861971848975944));
#19653=CARTESIAN_POINT('Ctrl Pts',(-1.01837060663223,-0.244234834628584,
0.0430711894098825));
#19654=CARTESIAN_POINT('Ctrl Pts',(-1.019052,-0.246942143572133,0.0206568624125608));
#19655=CARTESIAN_POINT('Ctrl Pts',(-1.019052,-0.246942143572133,1.2490009027033E-16));
#19656=CARTESIAN_POINT('',(-1.019052,-0.28578,1.24797876996471E-16));
#19657=CARTESIAN_POINT('',(-1.019052,-0.166705,1.24797876996471E-16));
#19658=CARTESIAN_POINT('Origin',(0.,-0.28578,0.));
#19659=CARTESIAN_POINT('',(-0.989696097314,-0.04763,-0.242834539687906));
#19660=CARTESIAN_POINT('Ctrl Pts',(-1.019052,-0.246942143572133,1.2490009027033E-16));
#19661=CARTESIAN_POINT('Ctrl Pts',(-1.019052,-0.246942143572133,-0.0206568624125605));
#19662=CARTESIAN_POINT('Ctrl Pts',(-1.01837060663223,-0.244234834628584,
-0.0430711894098822));
#19663=CARTESIAN_POINT('Ctrl Pts',(-1.0156297872271,-0.232742381310829,
-0.0861971848975941));
#19664=CARTESIAN_POINT('Ctrl Pts',(-1.01358704779679,-0.223955109275652,
-0.106909345252087));
#19665=CARTESIAN_POINT('Ctrl Pts',(-1.00869718865384,-0.201072148666546,
-0.1465689792446));
#19666=CARTESIAN_POINT('Ctrl Pts',(-1.00492400591205,-0.181890537957859,
-0.169940289819232));
#19667=CARTESIAN_POINT('Ctrl Pts',(-0.998375294985966,-0.141695629206859,
-0.205111543747588));
#19668=CARTESIAN_POINT('Ctrl Pts',(-0.994830026707808,-0.11549207705665,
-0.221129100087819));
#19669=CARTESIAN_POINT('Ctrl Pts',(-0.991238884025248,-0.0742967091364495,
-0.236509675094874));
#19670=CARTESIAN_POINT('Ctrl Pts',(-0.990332542620729,-0.0609922781173484,
-0.24024064412003));
#19671=CARTESIAN_POINT('Ctrl Pts',(-0.989696097314,-0.0476300000000001,
-0.242834539687907));
#19672=CARTESIAN_POINT('',(-0.871530771444223,-0.04763,-0.528110872004958));
#19673=CARTESIAN_POINT('Origin',(0.,-0.04763,0.));
#19674=CARTESIAN_POINT('',(-0.528110872004958,-0.04763,-0.871530771444223));
#19675=CARTESIAN_POINT('Ctrl Pts',(-0.871530771444223,-0.0476300000000001,
-0.528110872004958));
#19676=CARTESIAN_POINT('Ctrl Pts',(-0.87014664509073,-0.0609922781173484,
-0.530395067942936));
#19677=CARTESIAN_POINT('Ctrl Pts',(-0.868149331745851,-0.0742967091364494,
-0.533674141594226));
#19678=CARTESIAN_POINT('Ctrl Pts',(-0.85981294420286,-0.115492077056649,
-0.54708917182331));
#19679=CARTESIAN_POINT('Ctrl Pts',(-0.850993704737257,-0.141695629206859,
-0.560922177770136));
#19680=CARTESIAN_POINT('Ctrl Pts',(-0.830754510485543,-0.181890537957859,
-0.590422647829571));
#19681=CARTESIAN_POINT('Ctrl Pts',(-0.816896541396381,-0.201072148666546,
-0.609616703125488));
#19682=CARTESIAN_POINT('Ctrl Pts',(-0.792310597819928,-0.223955109275652,
-0.641117951819999));
#19683=CARTESIAN_POINT('Ctrl Pts',(-0.779109323683611,-0.232742381310829,
-0.657208095763053));
#19684=CARTESIAN_POINT('Ctrl Pts',(-0.750552691816205,-0.244234834628584,
-0.68964083160521));
#19685=CARTESIAN_POINT('Ctrl Pts',(-0.735185187071673,-0.246942143572133,
-0.705971972091755));
#19686=CARTESIAN_POINT('Ctrl Pts',(-0.705971972091754,-0.246942143572133,
-0.735185187071673));
#19687=CARTESIAN_POINT('Ctrl Pts',(-0.68964083160521,-0.244234834628584,
-0.750552691816206));
#19688=CARTESIAN_POINT('Ctrl Pts',(-0.657208095763052,-0.232742381310829,
-0.779109323683612));
#19689=CARTESIAN_POINT('Ctrl Pts',(-0.641117951819998,-0.223955109275652,
-0.792310597819928));
#19690=CARTESIAN_POINT('Ctrl Pts',(-0.609616703125488,-0.201072148666545,
-0.816896541396381));
#19691=CARTESIAN_POINT('Ctrl Pts',(-0.590422647829571,-0.181890537957859,
-0.830754510485543));
#19692=CARTESIAN_POINT('Ctrl Pts',(-0.560922177770136,-0.141695629206859,
-0.850993704737257));
#19693=CARTESIAN_POINT('Ctrl Pts',(-0.54708917182331,-0.115492077056649,
-0.85981294420286));
#19694=CARTESIAN_POINT('Ctrl Pts',(-0.533674141594226,-0.0742967091364494,
-0.868149331745852));
#19695=CARTESIAN_POINT('Ctrl Pts',(-0.530395067942936,-0.0609922781173484,
-0.870146645090731));
#19696=CARTESIAN_POINT('Ctrl Pts',(-0.528110872004958,-0.0476300000000001,
-0.871530771444223));
#19697=CARTESIAN_POINT('',(-0.242834539687906,-0.04763,-0.989696097314));
#19698=CARTESIAN_POINT('Origin',(0.,-0.04763,0.));
#19699=CARTESIAN_POINT('',(0.242834539687906,-0.04763,-0.989696097314));
#19700=CARTESIAN_POINT('Ctrl Pts',(-0.242834539687907,-0.04763,-0.989696097314));
#19701=CARTESIAN_POINT('Ctrl Pts',(-0.24024064412003,-0.0609922781173483,
-0.990332542620729));
#19702=CARTESIAN_POINT('Ctrl Pts',(-0.236509675094874,-0.0742967091364493,
-0.991238884025248));
#19703=CARTESIAN_POINT('Ctrl Pts',(-0.221129100087819,-0.115492077056649,
-0.994830026707808));
#19704=CARTESIAN_POINT('Ctrl Pts',(-0.205111543747588,-0.141695629206859,
-0.998375294985966));
#19705=CARTESIAN_POINT('Ctrl Pts',(-0.169940289819232,-0.181890537957859,
-1.00492400591205));
#19706=CARTESIAN_POINT('Ctrl Pts',(-0.1465689792446,-0.201072148666545,
-1.00869718865384));
#19707=CARTESIAN_POINT('Ctrl Pts',(-0.106909345252087,-0.223955109275652,
-1.01358704779679));
#19708=CARTESIAN_POINT('Ctrl Pts',(-0.0861971848975942,-0.232742381310829,
-1.0156297872271));
#19709=CARTESIAN_POINT('Ctrl Pts',(-0.0430711894098823,-0.244234834628584,
-1.01837060663223));
#19710=CARTESIAN_POINT('Ctrl Pts',(-0.0206568624125606,-0.246942143572133,
-1.019052));
#19711=CARTESIAN_POINT('Ctrl Pts',(0.0206568624125607,-0.246942143572133,
-1.019052));
#19712=CARTESIAN_POINT('Ctrl Pts',(0.0430711894098824,-0.244234834628584,
-1.01837060663223));
#19713=CARTESIAN_POINT('Ctrl Pts',(0.0861971848975943,-0.232742381310829,
-1.0156297872271));
#19714=CARTESIAN_POINT('Ctrl Pts',(0.106909345252088,-0.223955109275652,
-1.01358704779679));
#19715=CARTESIAN_POINT('Ctrl Pts',(0.1465689792446,-0.201072148666545,-1.00869718865384));
#19716=CARTESIAN_POINT('Ctrl Pts',(0.169940289819232,-0.181890537957859,
-1.00492400591205));
#19717=CARTESIAN_POINT('Ctrl Pts',(0.205111543747588,-0.141695629206859,
-0.998375294985966));
#19718=CARTESIAN_POINT('Ctrl Pts',(0.221129100087819,-0.115492077056649,
-0.994830026707808));
#19719=CARTESIAN_POINT('Ctrl Pts',(0.236509675094874,-0.0742967091364493,
-0.991238884025248));
#19720=CARTESIAN_POINT('Ctrl Pts',(0.24024064412003,-0.0609922781173484,
-0.990332542620729));
#19721=CARTESIAN_POINT('Ctrl Pts',(0.242834539687907,-0.04763,-0.989696097314));
#19722=CARTESIAN_POINT('',(0.528110872004958,-0.04763,-0.871530771444223));
#19723=CARTESIAN_POINT('Origin',(0.,-0.04763,0.));
#19724=CARTESIAN_POINT('',(0.871530771444223,-0.04763,-0.528110872004958));
#19725=CARTESIAN_POINT('Ctrl Pts',(0.528110872004958,-0.0476300000000001,
-0.871530771444223));
#19726=CARTESIAN_POINT('Ctrl Pts',(0.530395067942936,-0.0609922781173484,
-0.870146645090731));
#19727=CARTESIAN_POINT('Ctrl Pts',(0.533674141594226,-0.0742967091364493,
-0.868149331745851));
#19728=CARTESIAN_POINT('Ctrl Pts',(0.54708917182331,-0.115492077056649,
-0.85981294420286));
#19729=CARTESIAN_POINT('Ctrl Pts',(0.560922177770136,-0.141695629206859,
-0.850993704737257));
#19730=CARTESIAN_POINT('Ctrl Pts',(0.590422647829571,-0.181890537957859,
-0.830754510485543));
#19731=CARTESIAN_POINT('Ctrl Pts',(0.609616703125488,-0.201072148666545,
-0.816896541396381));
#19732=CARTESIAN_POINT('Ctrl Pts',(0.641117951819998,-0.223955109275652,
-0.792310597819928));
#19733=CARTESIAN_POINT('Ctrl Pts',(0.657208095763053,-0.232742381310829,
-0.779109323683612));
#19734=CARTESIAN_POINT('Ctrl Pts',(0.68964083160521,-0.244234834628584,
-0.750552691816206));
#19735=CARTESIAN_POINT('Ctrl Pts',(0.705971972091755,-0.246942143572133,
-0.735185187071673));
#19736=CARTESIAN_POINT('Ctrl Pts',(0.735185187071673,-0.246942143572133,
-0.705971972091754));
#19737=CARTESIAN_POINT('Ctrl Pts',(0.750552691816206,-0.244234834628584,
-0.68964083160521));
#19738=CARTESIAN_POINT('Ctrl Pts',(0.779109323683612,-0.232742381310829,
-0.657208095763053));
#19739=CARTESIAN_POINT('Ctrl Pts',(0.792310597819928,-0.223955109275652,
-0.641117951819998));
#19740=CARTESIAN_POINT('Ctrl Pts',(0.816896541396381,-0.201072148666545,
-0.609616703125488));
#19741=CARTESIAN_POINT('Ctrl Pts',(0.830754510485543,-0.181890537957859,
-0.590422647829571));
#19742=CARTESIAN_POINT('Ctrl Pts',(0.850993704737257,-0.141695629206859,
-0.560922177770136));
#19743=CARTESIAN_POINT('Ctrl Pts',(0.85981294420286,-0.115492077056649,
-0.54708917182331));
#19744=CARTESIAN_POINT('Ctrl Pts',(0.868149331745851,-0.0742967091364493,
-0.533674141594226));
#19745=CARTESIAN_POINT('Ctrl Pts',(0.870146645090731,-0.0609922781173484,
-0.530395067942936));
#19746=CARTESIAN_POINT('Ctrl Pts',(0.871530771444223,-0.0476300000000001,
-0.528110872004958));
#19747=CARTESIAN_POINT('',(0.989696097314,-0.04763,-0.242834539687906));
#19748=CARTESIAN_POINT('Origin',(0.,-0.04763,0.));
#19749=CARTESIAN_POINT('',(0.989696097314,-0.04763,0.242834539687906));
#19750=CARTESIAN_POINT('Ctrl Pts',(0.989696097314,-0.04763,-0.242834539687907));
#19751=CARTESIAN_POINT('Ctrl Pts',(0.990332542620729,-0.0609922781173483,
-0.24024064412003));
#19752=CARTESIAN_POINT('Ctrl Pts',(0.991238884025248,-0.0742967091364493,
-0.236509675094874));
#19753=CARTESIAN_POINT('Ctrl Pts',(0.994830026707808,-0.115492077056649,
-0.221129100087819));
#19754=CARTESIAN_POINT('Ctrl Pts',(0.998375294985966,-0.141695629206859,
-0.205111543747588));
#19755=CARTESIAN_POINT('Ctrl Pts',(1.00492400591205,-0.181890537957859,
-0.169940289819232));
#19756=CARTESIAN_POINT('Ctrl Pts',(1.00869718865384,-0.201072148666545,
-0.1465689792446));
#19757=CARTESIAN_POINT('Ctrl Pts',(1.01358704779679,-0.223955109275652,
-0.106909345252087));
#19758=CARTESIAN_POINT('Ctrl Pts',(1.0156297872271,-0.232742381310829,-0.0861971848975942));
#19759=CARTESIAN_POINT('Ctrl Pts',(1.01837060663223,-0.244234834628584,
-0.0430711894098823));
#19760=CARTESIAN_POINT('Ctrl Pts',(1.019052,-0.246942143572133,-0.0206568624125607));
#19761=CARTESIAN_POINT('Ctrl Pts',(1.019052,-0.246942143572133,0.0206568624125607));
#19762=CARTESIAN_POINT('Ctrl Pts',(1.01837060663223,-0.244234834628584,
0.0430711894098823));
#19763=CARTESIAN_POINT('Ctrl Pts',(1.0156297872271,-0.232742381310829,0.0861971848975942));
#19764=CARTESIAN_POINT('Ctrl Pts',(1.01358704779679,-0.223955109275652,
0.106909345252087));
#19765=CARTESIAN_POINT('Ctrl Pts',(1.00869718865384,-0.201072148666545,
0.1465689792446));
#19766=CARTESIAN_POINT('Ctrl Pts',(1.00492400591205,-0.181890537957859,
0.169940289819232));
#19767=CARTESIAN_POINT('Ctrl Pts',(0.998375294985966,-0.141695629206859,
0.205111543747588));
#19768=CARTESIAN_POINT('Ctrl Pts',(0.994830026707808,-0.115492077056649,
0.221129100087819));
#19769=CARTESIAN_POINT('Ctrl Pts',(0.991238884025248,-0.0742967091364492,
0.236509675094874));
#19770=CARTESIAN_POINT('Ctrl Pts',(0.990332542620729,-0.0609922781173483,
0.24024064412003));
#19771=CARTESIAN_POINT('Ctrl Pts',(0.989696097314,-0.04763,0.242834539687907));
#19772=CARTESIAN_POINT('Origin',(0.,-0.04763,0.));
#19773=CARTESIAN_POINT('Origin',(0.,-0.04763,0.));
#19774=CARTESIAN_POINT('',(0.238183666596899,-0.04763,0.951592097314));
#19775=CARTESIAN_POINT('Origin',(0.,-0.04763,0.));
#19776=CARTESIAN_POINT('Origin',(-1.94289029309402E-16,-0.04763,1.));
#19777=CARTESIAN_POINT('Origin',(-1.94289029309402E-16,0.,1.));
#19778=CARTESIAN_POINT('',(-0.2381836665969,-0.04763,0.951592097314));
#19779=CARTESIAN_POINT('Ctrl Pts',(-0.238183666596899,-0.0476299999999999,
0.951592097314));
#19780=CARTESIAN_POINT('Ctrl Pts',(-0.233157223576062,-0.0740444353928835,
0.952850216871763));
#19781=CARTESIAN_POINT('Ctrl Pts',(-0.223801617934946,-0.0999305678883309,
0.955173119738174));
#19782=CARTESIAN_POINT('Ctrl Pts',(-0.199966927975188,-0.142345102874864,
0.960411259488514));
#19783=CARTESIAN_POINT('Ctrl Pts',(-0.1868781821531,-0.159766064500479,
0.963103647174702));
#19784=CARTESIAN_POINT('Ctrl Pts',(-0.15681442133453,-0.190326085855194,
0.968453058988463));
#19785=CARTESIAN_POINT('Ctrl Pts',(-0.139836317888043,-0.203463743702801,
0.971100730005489));
#19786=CARTESIAN_POINT('Ctrl Pts',(-0.104422493053067,-0.224161999508995,
0.975530745318961));
#19787=CARTESIAN_POINT('Ctrl Pts',(-0.0842175114474176,-0.232861760990032,
0.977553872336861));
#19788=CARTESIAN_POINT('Ctrl Pts',(-0.0421062857595701,-0.244251601209411,
0.980270995488453));
#19789=CARTESIAN_POINT('Ctrl Pts',(-0.0201990724523197,-0.246942143572133,
0.980948));
#19790=CARTESIAN_POINT('Ctrl Pts',(0.020199072452319,-0.246942143572133,
0.980948));
#19791=CARTESIAN_POINT('Ctrl Pts',(0.0421062857595694,-0.244251601209411,
0.980270995488454));
#19792=CARTESIAN_POINT('Ctrl Pts',(0.0842175114474169,-0.232861760990032,
0.977553872336861));
#19793=CARTESIAN_POINT('Ctrl Pts',(0.104422493053067,-0.224161999508995,
0.975530745318961));
#19794=CARTESIAN_POINT('Ctrl Pts',(0.139836317888042,-0.203463743702801,
0.971100730005489));
#19795=CARTESIAN_POINT('Ctrl Pts',(0.15681442133453,-0.190326085855194,
0.968453058988463));
#19796=CARTESIAN_POINT('Ctrl Pts',(0.1868781821531,-0.15976606450048,0.963103647174702));
#19797=CARTESIAN_POINT('Ctrl Pts',(0.199966927975188,-0.142345102874864,
0.960411259488514));
#19798=CARTESIAN_POINT('Ctrl Pts',(0.223801617934945,-0.0999305678883309,
0.955173119738174));
#19799=CARTESIAN_POINT('Ctrl Pts',(0.233157223576061,-0.0740444353928835,
0.952850216871763));
#19800=CARTESIAN_POINT('Ctrl Pts',(0.238183666596899,-0.0476299999999999,
0.951592097314));
#19801=CARTESIAN_POINT('Origin',(-1.94289029309402E-16,-0.04763,1.));
#19802=CARTESIAN_POINT('Origin',(0.,-0.04763,0.));
#19803=CARTESIAN_POINT('',(-0.504455939115715,-0.04763,0.841298510752802));
#19804=CARTESIAN_POINT('Origin',(0.,-0.04763,0.));
#19805=CARTESIAN_POINT('Origin',(-0.707106781186548,-0.04763,0.707106781186547));
#19806=CARTESIAN_POINT('Origin',(-0.707106781186548,0.,0.707106781186547));
#19807=CARTESIAN_POINT('',(-0.841298510752802,-0.04763,0.504455939115715));
#19808=CARTESIAN_POINT('Ctrl Pts',(-0.841298510752802,-0.04763,0.504455939115715));
#19809=CARTESIAN_POINT('Ctrl Pts',(-0.838633903678357,-0.0740444353928835,
0.508899795931835));
#19810=CARTESIAN_POINT('Ctrl Pts',(-0.833661031856294,-0.0999305678883309,
0.517157748491652));
#19811=CARTESIAN_POINT('Ctrl Pts',(-0.820511285096538,-0.142345102874864,
0.537715343527944));
#19812=CARTESIAN_POINT('Ctrl Pts',(-0.813159949759,-0.159766064500479,0.548874290046456));
#19813=CARTESIAN_POINT('Ctrl Pts',(-0.795684265985089,-0.190326085855194,
0.573915184558107));
#19814=CARTESIAN_POINT('Ctrl Pts',(-0.78555112003688,-0.203463743702801,
0.587792702767295));
#19815=CARTESIAN_POINT('Ctrl Pts',(-0.763642258217233,-0.224161999508995,
0.615966552324775));
#19816=CARTESIAN_POINT('Ctrl Pts',(-0.750785745543687,-0.232861760990032,
0.631684198665438));
#19817=CARTESIAN_POINT('Ctrl Pts',(-0.722929908501543,-0.244251601209411,
0.663382628119203));
#19818=CARTESIAN_POINT('Ctrl Pts',(-0.707917883896095,-0.246942143572133,
0.679352081686668));
#19819=CARTESIAN_POINT('Ctrl Pts',(-0.679352081686668,-0.246942143572133,
0.707917883896095));
#19820=CARTESIAN_POINT('Ctrl Pts',(-0.663382628119203,-0.244251601209411,
0.722929908501544));
#19821=CARTESIAN_POINT('Ctrl Pts',(-0.631684198665438,-0.232861760990031,
0.750785745543687));
#19822=CARTESIAN_POINT('Ctrl Pts',(-0.615966552324775,-0.224161999508995,
0.763642258217233));
#19823=CARTESIAN_POINT('Ctrl Pts',(-0.587792702767295,-0.203463743702801,
0.78555112003688));
#19824=CARTESIAN_POINT('Ctrl Pts',(-0.573915184558107,-0.190326085855194,
0.795684265985088));
#19825=CARTESIAN_POINT('Ctrl Pts',(-0.548874290046456,-0.159766064500479,
0.813159949759));
#19826=CARTESIAN_POINT('Ctrl Pts',(-0.537715343527944,-0.142345102874864,
0.820511285096538));
#19827=CARTESIAN_POINT('Ctrl Pts',(-0.517157748491652,-0.0999305678883309,
0.833661031856294));
#19828=CARTESIAN_POINT('Ctrl Pts',(-0.508899795931835,-0.0740444353928835,
0.838633903678357));
#19829=CARTESIAN_POINT('Ctrl Pts',(-0.504455939115716,-0.04763,0.841298510752801));
#19830=CARTESIAN_POINT('Origin',(-0.707106781186548,-0.04763,0.707106781186547));
#19831=CARTESIAN_POINT('Origin',(0.,-0.04763,0.));
#19832=CARTESIAN_POINT('',(-0.951592097314,-0.04763,0.238183666596899));
#19833=CARTESIAN_POINT('Origin',(0.,-0.04763,0.));
#19834=CARTESIAN_POINT('Origin',(-1.,-0.04763,-1.11022302462516E-16));
#19835=CARTESIAN_POINT('Origin',(-1.,0.,-1.11022302462516E-16));
#19836=CARTESIAN_POINT('',(-0.951592097314,-0.04763,-0.2381836665969));
#19837=CARTESIAN_POINT('',(-0.980948,-0.246942143572133,1.08514323328844E-18));
#19838=CARTESIAN_POINT('Ctrl Pts',(-0.951592097314,-0.04763,-0.238183666596899));
#19839=CARTESIAN_POINT('Ctrl Pts',(-0.952850216871763,-0.0740444353928835,
-0.233157223576062));
#19840=CARTESIAN_POINT('Ctrl Pts',(-0.955173119738174,-0.0999305678883309,
-0.223801617934946));
#19841=CARTESIAN_POINT('Ctrl Pts',(-0.960411259488514,-0.142345102874864,
-0.199966927975188));
#19842=CARTESIAN_POINT('Ctrl Pts',(-0.963103647174702,-0.159766064500479,
-0.1868781821531));
#19843=CARTESIAN_POINT('Ctrl Pts',(-0.968453058988463,-0.190326085855194,
-0.15681442133453));
#19844=CARTESIAN_POINT('Ctrl Pts',(-0.971100730005489,-0.203463743702801,
-0.139836317888043));
#19845=CARTESIAN_POINT('Ctrl Pts',(-0.975530745318961,-0.224161999508995,
-0.104422493053067));
#19846=CARTESIAN_POINT('Ctrl Pts',(-0.977553872336861,-0.232861760990032,
-0.0842175114474175));
#19847=CARTESIAN_POINT('Ctrl Pts',(-0.980270995488453,-0.244251601209411,
-0.0421062857595699));
#19848=CARTESIAN_POINT('Ctrl Pts',(-0.980948,-0.246942143572133,-0.0201990724523195));
#19849=CARTESIAN_POINT('Ctrl Pts',(-0.980948,-0.246942143572133,-1.17961196366423E-16));
#19850=CARTESIAN_POINT('Origin',(-1.,-0.04763,-1.11022302462516E-16));
#19851=CARTESIAN_POINT('Ctrl Pts',(-0.980948,-0.246942143572133,-1.17961196366423E-16));
#19852=CARTESIAN_POINT('Ctrl Pts',(-0.980948,-0.246942143572133,0.0201990724523192));
#19853=CARTESIAN_POINT('Ctrl Pts',(-0.980270995488453,-0.244251601209411,
0.0421062857595695));
#19854=CARTESIAN_POINT('Ctrl Pts',(-0.977553872336861,-0.232861760990032,
0.0842175114474169));
#19855=CARTESIAN_POINT('Ctrl Pts',(-0.975530745318961,-0.224161999508995,
0.104422493053066));
#19856=CARTESIAN_POINT('Ctrl Pts',(-0.971100730005489,-0.203463743702801,
0.139836317888042));
#19857=CARTESIAN_POINT('Ctrl Pts',(-0.968453058988463,-0.190326085855194,
0.15681442133453));
#19858=CARTESIAN_POINT('Ctrl Pts',(-0.963103647174702,-0.15976606450048,
0.1868781821531));
#19859=CARTESIAN_POINT('Ctrl Pts',(-0.960411259488514,-0.142345102874864,
0.199966927975188));
#19860=CARTESIAN_POINT('Ctrl Pts',(-0.955173119738174,-0.099930567888331,
0.223801617934945));
#19861=CARTESIAN_POINT('Ctrl Pts',(-0.952850216871763,-0.0740444353928835,
0.233157223576061));
#19862=CARTESIAN_POINT('Ctrl Pts',(-0.951592097314,-0.04763,0.238183666596899));
#19863=CARTESIAN_POINT('Origin',(0.,-0.04763,0.));
#19864=CARTESIAN_POINT('',(-0.841298510752802,-0.04763,-0.504455939115715));
#19865=CARTESIAN_POINT('Origin',(0.,-0.04763,0.));
#19866=CARTESIAN_POINT('Origin',(-0.707106781186547,-0.04763,-0.707106781186548));
#19867=CARTESIAN_POINT('Origin',(-0.707106781186547,0.,-0.707106781186548));
#19868=CARTESIAN_POINT('',(-0.504455939115715,-0.04763,-0.841298510752802));
#19869=CARTESIAN_POINT('Ctrl Pts',(-0.504455939115715,-0.04763,-0.841298510752802));
#19870=CARTESIAN_POINT('Ctrl Pts',(-0.508899795931835,-0.0740444353928835,
-0.838633903678357));
#19871=CARTESIAN_POINT('Ctrl Pts',(-0.517157748491652,-0.0999305678883309,
-0.833661031856294));
#19872=CARTESIAN_POINT('Ctrl Pts',(-0.537715343527944,-0.142345102874864,
-0.820511285096538));
#19873=CARTESIAN_POINT('Ctrl Pts',(-0.548874290046456,-0.159766064500479,
-0.813159949759));
#19874=CARTESIAN_POINT('Ctrl Pts',(-0.573915184558107,-0.190326085855194,
-0.795684265985089));
#19875=CARTESIAN_POINT('Ctrl Pts',(-0.587792702767295,-0.203463743702801,
-0.78555112003688));
#19876=CARTESIAN_POINT('Ctrl Pts',(-0.615966552324775,-0.224161999508995,
-0.763642258217233));
#19877=CARTESIAN_POINT('Ctrl Pts',(-0.631684198665438,-0.232861760990032,
-0.750785745543687));
#19878=CARTESIAN_POINT('Ctrl Pts',(-0.663382628119203,-0.244251601209411,
-0.722929908501543));
#19879=CARTESIAN_POINT('Ctrl Pts',(-0.679352081686668,-0.246942143572133,
-0.707917883896095));
#19880=CARTESIAN_POINT('Ctrl Pts',(-0.707917883896095,-0.246942143572133,
-0.679352081686668));
#19881=CARTESIAN_POINT('Ctrl Pts',(-0.722929908501543,-0.244251601209411,
-0.663382628119203));
#19882=CARTESIAN_POINT('Ctrl Pts',(-0.750785745543687,-0.232861760990032,
-0.631684198665439));
#19883=CARTESIAN_POINT('Ctrl Pts',(-0.763642258217232,-0.224161999508995,
-0.615966552324775));
#19884=CARTESIAN_POINT('Ctrl Pts',(-0.78555112003688,-0.203463743702801,
-0.587792702767295));
#19885=CARTESIAN_POINT('Ctrl Pts',(-0.795684265985088,-0.190326085855194,
-0.573915184558107));
#19886=CARTESIAN_POINT('Ctrl Pts',(-0.813159949759,-0.15976606450048,-0.548874290046456));
#19887=CARTESIAN_POINT('Ctrl Pts',(-0.820511285096538,-0.142345102874864,
-0.537715343527944));
#19888=CARTESIAN_POINT('Ctrl Pts',(-0.833661031856294,-0.0999305678883311,
-0.517157748491652));
#19889=CARTESIAN_POINT('Ctrl Pts',(-0.838633903678357,-0.0740444353928836,
-0.508899795931835));
#19890=CARTESIAN_POINT('Ctrl Pts',(-0.841298510752801,-0.04763,-0.504455939115715));
#19891=CARTESIAN_POINT('Origin',(-0.707106781186547,-0.04763,-0.707106781186548));
#19892=CARTESIAN_POINT('Origin',(0.,-0.04763,0.));
#19893=CARTESIAN_POINT('',(-0.238183666596899,-0.04763,-0.951592097314));
#19894=CARTESIAN_POINT('Origin',(0.,-0.04763,0.));
#19895=CARTESIAN_POINT('Origin',(5.55111512312578E-17,-0.04763,-1.));
#19896=CARTESIAN_POINT('Origin',(5.55111512312578E-17,0.,-1.));
#19897=CARTESIAN_POINT('',(0.238183666596899,-0.04763,-0.951592097314));
#19898=CARTESIAN_POINT('Ctrl Pts',(0.238183666596899,-0.04763,-0.951592097314));
#19899=CARTESIAN_POINT('Ctrl Pts',(0.233157223576062,-0.0740444353928835,
-0.952850216871763));
#19900=CARTESIAN_POINT('Ctrl Pts',(0.223801617934946,-0.099930567888331,
-0.955173119738174));
#19901=CARTESIAN_POINT('Ctrl Pts',(0.199966927975188,-0.142345102874864,
-0.960411259488514));
#19902=CARTESIAN_POINT('Ctrl Pts',(0.1868781821531,-0.15976606450048,-0.963103647174702));
#19903=CARTESIAN_POINT('Ctrl Pts',(0.15681442133453,-0.190326085855194,
-0.968453058988463));
#19904=CARTESIAN_POINT('Ctrl Pts',(0.139836317888042,-0.203463743702801,
-0.971100730005489));
#19905=CARTESIAN_POINT('Ctrl Pts',(0.104422493053067,-0.224161999508995,
-0.975530745318961));
#19906=CARTESIAN_POINT('Ctrl Pts',(0.0842175114474173,-0.232861760990032,
-0.977553872336861));
#19907=CARTESIAN_POINT('Ctrl Pts',(0.0421062857595698,-0.244251601209411,
-0.980270995488453));
#19908=CARTESIAN_POINT('Ctrl Pts',(0.0201990724523194,-0.246942143572133,
-0.980948));
#19909=CARTESIAN_POINT('Ctrl Pts',(-0.0201990724523193,-0.246942143572133,
-0.980948));
#19910=CARTESIAN_POINT('Ctrl Pts',(-0.0421062857595697,-0.244251601209411,
-0.980270995488453));
#19911=CARTESIAN_POINT('Ctrl Pts',(-0.0842175114474171,-0.232861760990032,
-0.977553872336861));
#19912=CARTESIAN_POINT('Ctrl Pts',(-0.104422493053067,-0.224161999508995,
-0.975530745318961));
#19913=CARTESIAN_POINT('Ctrl Pts',(-0.139836317888042,-0.203463743702801,
-0.971100730005489));
#19914=CARTESIAN_POINT('Ctrl Pts',(-0.15681442133453,-0.190326085855194,
-0.968453058988463));
#19915=CARTESIAN_POINT('Ctrl Pts',(-0.1868781821531,-0.15976606450048,-0.963103647174702));
#19916=CARTESIAN_POINT('Ctrl Pts',(-0.199966927975188,-0.142345102874864,
-0.960411259488514));
#19917=CARTESIAN_POINT('Ctrl Pts',(-0.223801617934945,-0.099930567888331,
-0.955173119738174));
#19918=CARTESIAN_POINT('Ctrl Pts',(-0.233157223576062,-0.0740444353928835,
-0.952850216871763));
#19919=CARTESIAN_POINT('Ctrl Pts',(-0.238183666596899,-0.0476299999999999,
-0.951592097314));
#19920=CARTESIAN_POINT('Origin',(5.55111512312578E-17,-0.04763,-1.));
#19921=CARTESIAN_POINT('Origin',(0.,-0.04763,0.));
#19922=CARTESIAN_POINT('',(0.504455939115715,-0.04763,-0.841298510752802));
#19923=CARTESIAN_POINT('Origin',(0.,-0.04763,0.));
#19924=CARTESIAN_POINT('Origin',(0.707106781186548,-0.04763,-0.707106781186547));
#19925=CARTESIAN_POINT('Origin',(0.707106781186548,0.,-0.707106781186547));
#19926=CARTESIAN_POINT('',(0.841298510752802,-0.04763,-0.504455939115715));
#19927=CARTESIAN_POINT('Ctrl Pts',(0.841298510752802,-0.04763,-0.504455939115715));
#19928=CARTESIAN_POINT('Ctrl Pts',(0.838633903678357,-0.0740444353928835,
-0.508899795931835));
#19929=CARTESIAN_POINT('Ctrl Pts',(0.833661031856294,-0.0999305678883309,
-0.517157748491652));
#19930=CARTESIAN_POINT('Ctrl Pts',(0.820511285096538,-0.142345102874864,
-0.537715343527944));
#19931=CARTESIAN_POINT('Ctrl Pts',(0.813159949759,-0.159766064500479,-0.548874290046456));
#19932=CARTESIAN_POINT('Ctrl Pts',(0.795684265985088,-0.190326085855194,
-0.573915184558107));
#19933=CARTESIAN_POINT('Ctrl Pts',(0.78555112003688,-0.203463743702801,
-0.587792702767295));
#19934=CARTESIAN_POINT('Ctrl Pts',(0.763642258217233,-0.224161999508995,
-0.615966552324775));
#19935=CARTESIAN_POINT('Ctrl Pts',(0.750785745543687,-0.232861760990032,
-0.631684198665438));
#19936=CARTESIAN_POINT('Ctrl Pts',(0.722929908501543,-0.244251601209411,
-0.663382628119203));
#19937=CARTESIAN_POINT('Ctrl Pts',(0.707917883896095,-0.246942143572133,
-0.679352081686668));
#19938=CARTESIAN_POINT('Ctrl Pts',(0.679352081686668,-0.246942143572133,
-0.707917883896095));
#19939=CARTESIAN_POINT('Ctrl Pts',(0.663382628119203,-0.244251601209411,
-0.722929908501543));
#19940=CARTESIAN_POINT('Ctrl Pts',(0.631684198665438,-0.232861760990032,
-0.750785745543687));
#19941=CARTESIAN_POINT('Ctrl Pts',(0.615966552324775,-0.224161999508995,
-0.763642258217232));
#19942=CARTESIAN_POINT('Ctrl Pts',(0.587792702767295,-0.203463743702801,
-0.78555112003688));
#19943=CARTESIAN_POINT('Ctrl Pts',(0.573915184558107,-0.190326085855194,
-0.795684265985088));
#19944=CARTESIAN_POINT('Ctrl Pts',(0.548874290046456,-0.159766064500479,
-0.813159949759));
#19945=CARTESIAN_POINT('Ctrl Pts',(0.537715343527944,-0.142345102874864,
-0.820511285096538));
#19946=CARTESIAN_POINT('Ctrl Pts',(0.517157748491652,-0.099930567888331,
-0.833661031856294));
#19947=CARTESIAN_POINT('Ctrl Pts',(0.508899795931835,-0.0740444353928835,
-0.838633903678357));
#19948=CARTESIAN_POINT('Ctrl Pts',(0.504455939115715,-0.04763,-0.841298510752801));
#19949=CARTESIAN_POINT('Origin',(0.707106781186548,-0.04763,-0.707106781186547));
#19950=CARTESIAN_POINT('Origin',(0.,-0.166705,0.));
#19951=CARTESIAN_POINT('',(-0.980948,-0.28578,1.20131482833E-16));
#19952=CARTESIAN_POINT('Origin',(0.,-0.28578,0.));
#19953=CARTESIAN_POINT('',(-0.980948,-0.166705,1.20131482833E-16));
#19954=CARTESIAN_POINT('',(0.951592097314,-0.04763,0.238183666596899));
#19955=CARTESIAN_POINT('Origin',(0.,-0.04763,0.));
#19956=CARTESIAN_POINT('',(0.951592097314,-0.04763,-0.238183666596899));
#19957=CARTESIAN_POINT('Ctrl Pts',(0.951592097314,-0.04763,0.238183666596899));
#19958=CARTESIAN_POINT('Ctrl Pts',(0.952850216871763,-0.0740444353928835,
0.233157223576062));
#19959=CARTESIAN_POINT('Ctrl Pts',(0.955173119738174,-0.099930567888331,
0.223801617934945));
#19960=CARTESIAN_POINT('Ctrl Pts',(0.960411259488514,-0.142345102874864,
0.199966927975188));
#19961=CARTESIAN_POINT('Ctrl Pts',(0.963103647174702,-0.15976606450048,
0.1868781821531));
#19962=CARTESIAN_POINT('Ctrl Pts',(0.968453058988463,-0.190326085855194,
0.15681442133453));
#19963=CARTESIAN_POINT('Ctrl Pts',(0.971100730005489,-0.203463743702801,
0.139836317888042));
#19964=CARTESIAN_POINT('Ctrl Pts',(0.975530745318961,-0.224161999508995,
0.104422493053067));
#19965=CARTESIAN_POINT('Ctrl Pts',(0.977553872336861,-0.232861760990032,
0.0842175114474172));
#19966=CARTESIAN_POINT('Ctrl Pts',(0.980270995488453,-0.244251601209411,
0.0421062857595697));
#19967=CARTESIAN_POINT('Ctrl Pts',(0.980948,-0.246942143572133,0.0201990724523194));
#19968=CARTESIAN_POINT('Ctrl Pts',(0.980948,-0.246942143572133,-0.0201990724523194));
#19969=CARTESIAN_POINT('Ctrl Pts',(0.980270995488453,-0.244251601209411,
-0.0421062857595697));
#19970=CARTESIAN_POINT('Ctrl Pts',(0.977553872336861,-0.232861760990032,
-0.0842175114474172));
#19971=CARTESIAN_POINT('Ctrl Pts',(0.975530745318961,-0.224161999508995,
-0.104422493053067));
#19972=CARTESIAN_POINT('Ctrl Pts',(0.971100730005489,-0.203463743702801,
-0.139836317888042));
#19973=CARTESIAN_POINT('Ctrl Pts',(0.968453058988463,-0.190326085855194,
-0.15681442133453));
#19974=CARTESIAN_POINT('Ctrl Pts',(0.963103647174702,-0.15976606450048,
-0.1868781821531));
#19975=CARTESIAN_POINT('Ctrl Pts',(0.960411259488514,-0.142345102874864,
-0.199966927975188));
#19976=CARTESIAN_POINT('Ctrl Pts',(0.955173119738174,-0.099930567888331,
-0.223801617934945));
#19977=CARTESIAN_POINT('Ctrl Pts',(0.952850216871763,-0.0740444353928835,
-0.233157223576062));
#19978=CARTESIAN_POINT('Ctrl Pts',(0.951592097314,-0.0476299999999999,-0.238183666596899));
#19979=CARTESIAN_POINT('Origin',(0.,-0.04763,0.));
#19980=CARTESIAN_POINT('Origin',(0.,-0.04763,0.));
#19981=CARTESIAN_POINT('Origin',(1.,-0.04763,0.));
#19982=CARTESIAN_POINT('Origin',(1.,0.,0.));
#19983=CARTESIAN_POINT('Origin',(1.,-0.04763,0.));
#19984=CARTESIAN_POINT('Origin',(0.,-0.28578,0.));
#19985=CARTESIAN_POINT('Origin',(0.,-0.04763,0.));
#23478=UNCERTAINTY_MEASURE_WITH_UNIT(LENGTH_MEASURE(0.001),#23588,
'DISTANCE_ACCURACY_VALUE',
'Maximum model space distance between geometric entities at asserted c
onnectivities');
#23522=UNCERTAINTY_MEASURE_WITH_UNIT(LENGTH_MEASURE(0.001),#23588,
'DISTANCE_ACCURACY_VALUE',
'Maximum model space distance between geometric entities at asserted c
onnectivities');
#23543=(
GEOMETRIC_REPRESENTATION_CONTEXT(3)
GLOBAL_UNCERTAINTY_ASSIGNED_CONTEXT((#23478))
GLOBAL_UNIT_ASSIGNED_CONTEXT((#23588,#23590,#23591))
REPRESENTATION_CONTEXT('','3D')
);
#23587=(
GEOMETRIC_REPRESENTATION_CONTEXT(3)
GLOBAL_UNCERTAINTY_ASSIGNED_CONTEXT((#23522))
GLOBAL_UNIT_ASSIGNED_CONTEXT((#23588,#23590,#23591))
REPRESENTATION_CONTEXT('','3D')
);
#23588=(
LENGTH_UNIT()
NAMED_UNIT(*)
SI_UNIT(.CENTI.,.METRE.)
);
#23590=(
NAMED_UNIT(*)
PLANE_ANGLE_UNIT()
SI_UNIT($,.RADIAN.)
);
#23591=(
NAMED_UNIT(*)
SI_UNIT($,.STERADIAN.)
SOLID_ANGLE_UNIT()
);
#23612=SHAPE_DEFINITION_REPRESENTATION(#23676,#23845);
#23676=PRODUCT_DEFINITION_SHAPE('',$,#23910);
#23845=SHAPE_REPRESENTATION('',(#13279),#23543);
#23889=PRODUCT_DEFINITION_CONTEXT('part definition',#24083,'design');
#23910=PRODUCT_DEFINITION('Cage','Cage',#23974,#23889);
#23974=PRODUCT_DEFINITION_FORMATION('',$,#24105);
#24083=APPLICATION_CONTEXT(
'Core Data for Automotive Mechanical Design Process');
#24084=PRODUCT_CONTEXT('part definition',#24083,'mechanical');
#24105=PRODUCT('Cage','Cage','Cage',(#24084));
#24205=COLOUR_RGB('Grey',0.48,0.52,0.57);
#24206=FILL_AREA_STYLE_COLOUR('',#24205);
#24207=FILL_AREA_STYLE('',(#24206));
#24208=SURFACE_STYLE_FILL_AREA(#24207);
#24209=SURFACE_SIDE_STYLE('',(#24208));
#24210=SURFACE_STYLE_USAGE(.BOTH.,#24209);
#24211=PRESENTATION_STYLE_ASSIGNMENT((#24210));
ENDSEC;
END-ISO-10303-21;
